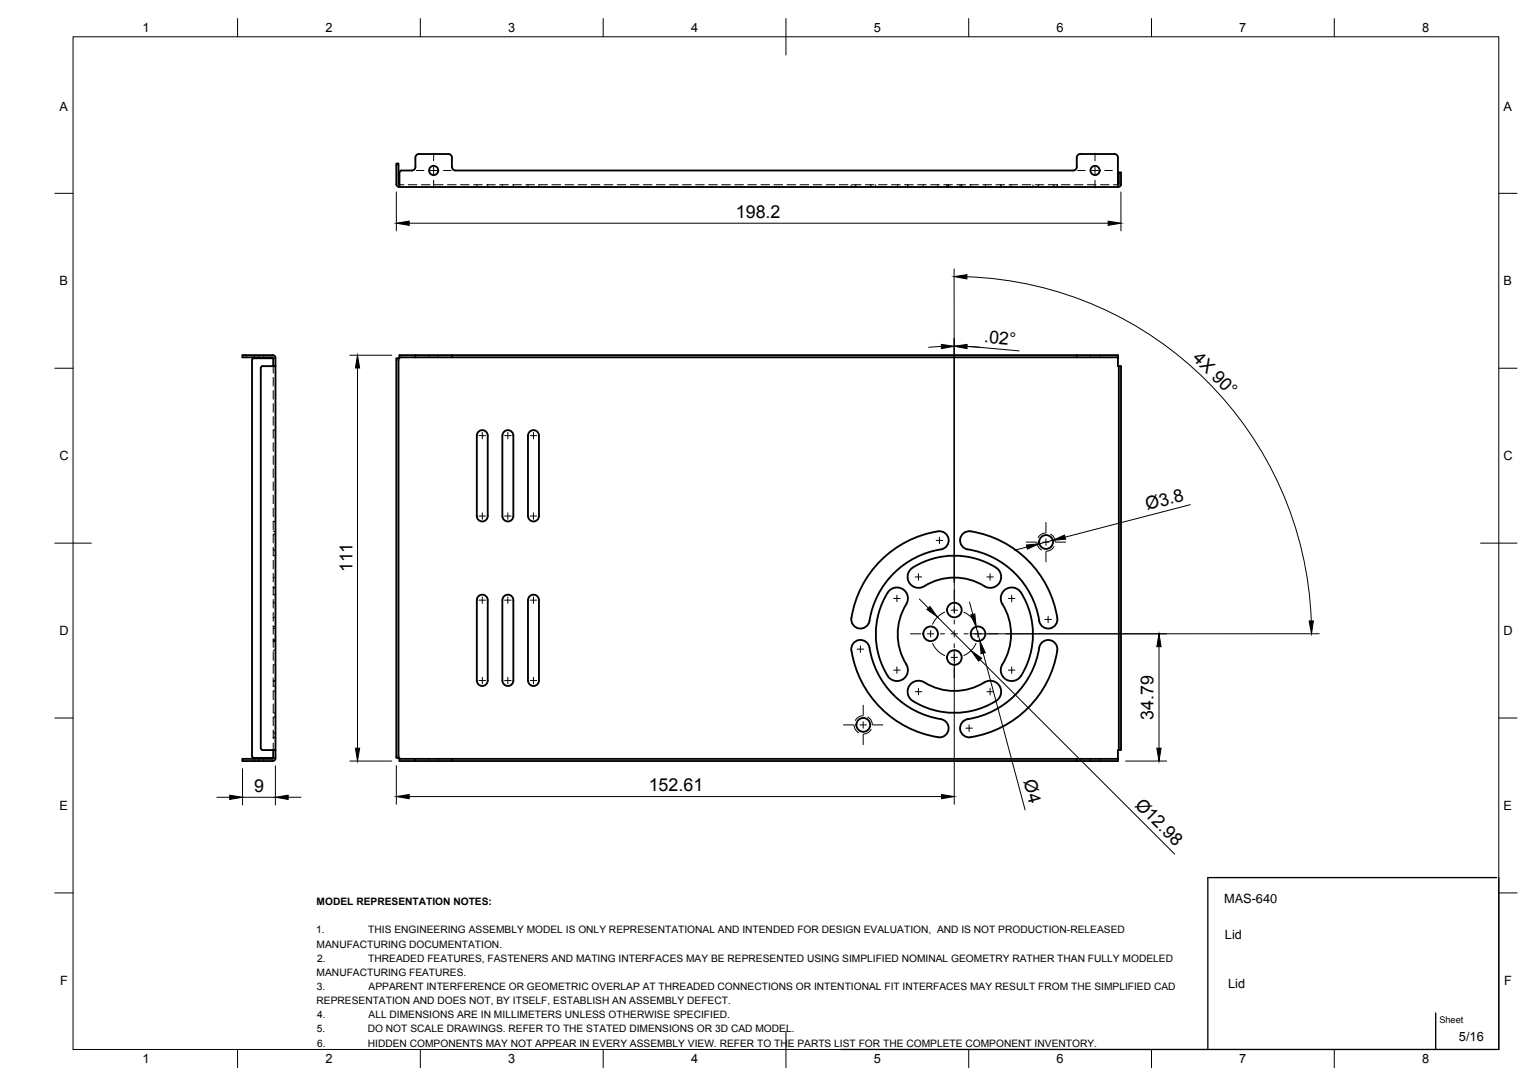
ISO-10303-21;
HEADER;
FILE_DESCRIPTION((''),'2;1');
FILE_NAME('Lid.step','2026-10-09T10:33:02-07:00',(''),(''),'','','');
FILE_SCHEMA (('AUTOMOTIVE_DESIGN { 1 0 10303 214 3 1 1 }'));
ENDSEC;
DATA;
#10=MECHANICAL_DESIGN_GEOMETRIC_PRESENTATION_REPRESENTATION('',(#838),#86330);
#814=SHAPE_REPRESENTATION_RELATIONSHIP('SRR','None',#86453,#826) ;
#826=ADVANCED_BREP_SHAPE_REPRESENTATION('',(#850),#86307) ;
#838=STYLED_ITEM('',(#86581),#850) ;
#850=MANIFOLD_SOLID_BREP('Body1',#32637) ;
#862=CONICAL_SURFACE('',#33010,2.390165042945,0.785398163397448) ;
#863=CONICAL_SURFACE('',#33011,2.390165042945,0.785398163397448) ;
#903=B_SPLINE_SURFACE_WITH_KNOTS('',3,3,((#46889,#46890,#46891,#46892),
(#46893,#46894,#46895,#46896),(#46897,#46898,#46899,#46900),(#46901,#46902,
#46903,#46904),(#46905,#46906,#46907,#46908),(#46909,#46910,#46911,#46912),
(#46913,#46914,#46915,#46916)),.UNSPECIFIED.,.F.,.F.,.F.,(4,1,1,1,4),(4,
4),(0.,0.285714285714286,0.571428571428571,0.857142857142857,1.),(0.250000208289045,
0.310000208302026),.UNSPECIFIED.) ;
#904=B_SPLINE_SURFACE_WITH_KNOTS('',3,3,((#46923,#46924,#46925,#46926),
(#46927,#46928,#46929,#46930),(#46931,#46932,#46933,#46934),(#46935,#46936,
#46937,#46938),(#46939,#46940,#46941,#46942),(#46943,#46944,#46945,#46946),
(#46947,#46948,#46949,#46950)),.UNSPECIFIED.,.F.,.F.,.F.,(4,1,1,1,4),(4,
4),(0.,0.285714285714286,0.571428571428571,0.857142857142857,1.),(-1.50824147057263E-10,
0.0600000000000031),.UNSPECIFIED.) ;
#1000=FACE_BOUND('',#4160,.T.) ;
#1001=FACE_BOUND('',#4161,.T.) ;
#1002=FACE_BOUND('',#4162,.T.) ;
#1003=FACE_BOUND('',#4163,.T.) ;
#1004=FACE_BOUND('',#4164,.T.) ;
#1005=FACE_BOUND('',#4165,.T.) ;
#1006=FACE_BOUND('',#4166,.T.) ;
#1007=FACE_BOUND('',#4167,.T.) ;
#1008=FACE_BOUND('',#4168,.T.) ;
#1009=FACE_BOUND('',#4169,.T.) ;
#1010=FACE_BOUND('',#4170,.T.) ;
#1011=FACE_BOUND('',#4171,.T.) ;
#1012=FACE_BOUND('',#4172,.T.) ;
#1013=FACE_BOUND('',#4173,.T.) ;
#1014=FACE_BOUND('',#4174,.T.) ;
#1015=FACE_BOUND('',#4175,.T.) ;
#1016=FACE_BOUND('',#4176,.T.) ;
#1017=FACE_BOUND('',#4177,.T.) ;
#1018=FACE_BOUND('',#4178,.T.) ;
#1019=FACE_BOUND('',#4179,.T.) ;
#1020=FACE_BOUND('',#4183,.T.) ;
#1021=FACE_BOUND('',#4184,.T.) ;
#1022=FACE_BOUND('',#4188,.T.) ;
#1023=FACE_BOUND('',#4189,.T.) ;
#1024=FACE_BOUND('',#4193,.T.) ;
#1025=FACE_BOUND('',#4194,.T.) ;
#1026=FACE_BOUND('',#4202,.T.) ;
#1027=FACE_BOUND('',#4203,.T.) ;
#1028=FACE_BOUND('',#4204,.T.) ;
#1029=FACE_BOUND('',#4205,.T.) ;
#1030=FACE_BOUND('',#4206,.T.) ;
#1031=FACE_BOUND('',#4207,.T.) ;
#1032=FACE_BOUND('',#4208,.T.) ;
#1033=FACE_BOUND('',#4209,.T.) ;
#1034=FACE_BOUND('',#4210,.T.) ;
#1035=FACE_BOUND('',#4211,.T.) ;
#1036=FACE_BOUND('',#4212,.T.) ;
#1037=FACE_BOUND('',#4213,.T.) ;
#1038=FACE_BOUND('',#4214,.T.) ;
#1039=FACE_BOUND('',#4215,.T.) ;
#1040=FACE_BOUND('',#4216,.T.) ;
#1041=FACE_BOUND('',#4217,.T.) ;
#1042=FACE_BOUND('',#4218,.T.) ;
#1043=FACE_BOUND('',#4219,.T.) ;
#1044=FACE_BOUND('',#4220,.T.) ;
#1045=FACE_BOUND('',#4221,.T.) ;
#1046=FACE_BOUND('',#4223,.T.) ;
#1047=FACE_BOUND('',#4224,.T.) ;
#1189=B_SPLINE_CURVE_WITH_KNOTS('',3,(#46372,#46373,#46374,#46375,#46376,
#46377,#46378),.UNSPECIFIED.,.F.,.F.,(4,1,1,1,4),(0.,0.112519573127489,
0.337558719382466,0.562597865637444,0.787637011892422),.UNSPECIFIED.) ;
#1190=B_SPLINE_CURVE_WITH_KNOTS('',3,(#46384,#46385,#46386,#46387,#46388,
#46389,#46390),.UNSPECIFIED.,.F.,.F.,(4,1,1,1,4),(0.,0.112518191393291,
0.337554574179873,0.562590956966454,0.787627339753036),.UNSPECIFIED.) ;
#1191=B_SPLINE_CURVE_WITH_KNOTS('',3,(#46817,#46818,#46819,#46820,#46821,
#46822,#46823),.UNSPECIFIED.,.F.,.F.,(4,1,1,1,4),(0.,0.22503638292787,0.45007276585574,
0.675109148783609,0.787627340247544),.UNSPECIFIED.) ;
#1192=B_SPLINE_CURVE_WITH_KNOTS('',3,(#46831,#46832,#46833,#46834,#46835,
#46836,#46837),.UNSPECIFIED.,.F.,.F.,(4,1,1,1,4),(0.,0.225039146153262,
0.450078292306524,0.675117438459786,0.787637011536417),.UNSPECIFIED.) ;
#1706=PLANE('',#32777) ;
#1707=PLANE('',#32832) ;
#1708=PLANE('',#32846) ;
#1709=PLANE('',#32847) ;
#1710=PLANE('',#32861) ;
#1711=PLANE('',#32862) ;
#1712=PLANE('',#32875) ;
#1713=PLANE('',#32877) ;
#1714=PLANE('',#32881) ;
#1715=PLANE('',#32882) ;
#1716=PLANE('',#32931) ;
#1717=PLANE('',#32941) ;
#1718=PLANE('',#32956) ;
#1719=PLANE('',#32959) ;
#1720=PLANE('',#32964) ;
#1721=PLANE('',#32965) ;
#1722=PLANE('',#32969) ;
#1723=PLANE('',#32973) ;
#1724=PLANE('',#32975) ;
#1725=PLANE('',#32977) ;
#1726=PLANE('',#32980) ;
#1727=PLANE('',#32982) ;
#1728=PLANE('',#32985) ;
#1729=PLANE('',#32987) ;
#1730=PLANE('',#32990) ;
#1731=PLANE('',#32992) ;
#1732=PLANE('',#32994) ;
#1733=PLANE('',#32997) ;
#1734=PLANE('',#32999) ;
#1735=PLANE('',#33000) ;
#1736=PLANE('',#33003) ;
#1737=PLANE('',#33012) ;
#1738=PLANE('',#33013) ;
#1739=PLANE('',#33019) ;
#1740=PLANE('',#33021) ;
#1741=PLANE('',#33023) ;
#1742=PLANE('',#33025) ;
#1743=PLANE('',#33027) ;
#1744=PLANE('',#33029) ;
#1745=PLANE('',#33031) ;
#1746=PLANE('',#33033) ;
#1747=PLANE('',#33035) ;
#1748=PLANE('',#33037) ;
#1749=PLANE('',#33039) ;
#1750=PLANE('',#33041) ;
#1751=PLANE('',#33043) ;
#2270=FACE_OUTER_BOUND('',#4158,.T.) ;
#2271=FACE_OUTER_BOUND('',#4159,.T.) ;
#2272=FACE_OUTER_BOUND('',#4180,.T.) ;
#2273=FACE_OUTER_BOUND('',#4181,.T.) ;
#2274=FACE_OUTER_BOUND('',#4182,.T.) ;
#2275=FACE_OUTER_BOUND('',#4185,.T.) ;
#2276=FACE_OUTER_BOUND('',#4186,.T.) ;
#2277=FACE_OUTER_BOUND('',#4187,.T.) ;
#2278=FACE_OUTER_BOUND('',#4190,.T.) ;
#2279=FACE_OUTER_BOUND('',#4191,.T.) ;
#2280=FACE_OUTER_BOUND('',#4192,.T.) ;
#2281=FACE_OUTER_BOUND('',#4195,.T.) ;
#2282=FACE_OUTER_BOUND('',#4196,.T.) ;
#2283=FACE_OUTER_BOUND('',#4197,.T.) ;
#2284=FACE_OUTER_BOUND('',#4198,.T.) ;
#2285=FACE_OUTER_BOUND('',#4199,.T.) ;
#2286=FACE_OUTER_BOUND('',#4200,.T.) ;
#2287=FACE_OUTER_BOUND('',#4201,.T.) ;
#2288=FACE_OUTER_BOUND('',#4222,.T.) ;
#2289=FACE_OUTER_BOUND('',#4225,.T.) ;
#2290=FACE_OUTER_BOUND('',#4226,.T.) ;
#2291=FACE_OUTER_BOUND('',#4227,.T.) ;
#2292=FACE_OUTER_BOUND('',#4228,.T.) ;
#2293=FACE_OUTER_BOUND('',#4229,.T.) ;
#2294=FACE_OUTER_BOUND('',#4230,.T.) ;
#2295=FACE_OUTER_BOUND('',#4231,.T.) ;
#2296=FACE_OUTER_BOUND('',#4232,.T.) ;
#2297=FACE_OUTER_BOUND('',#4233,.T.) ;
#2298=FACE_OUTER_BOUND('',#4234,.T.) ;
#2299=FACE_OUTER_BOUND('',#4235,.T.) ;
#2300=FACE_OUTER_BOUND('',#4236,.T.) ;
#2301=FACE_OUTER_BOUND('',#4237,.T.) ;
#2302=FACE_OUTER_BOUND('',#4238,.T.) ;
#2303=FACE_OUTER_BOUND('',#4239,.T.) ;
#2304=FACE_OUTER_BOUND('',#4240,.T.) ;
#2305=FACE_OUTER_BOUND('',#4241,.T.) ;
#2306=FACE_OUTER_BOUND('',#4242,.T.) ;
#2307=FACE_OUTER_BOUND('',#4243,.T.) ;
#2308=FACE_OUTER_BOUND('',#4244,.T.) ;
#2309=FACE_OUTER_BOUND('',#4245,.T.) ;
#2310=FACE_OUTER_BOUND('',#4246,.T.) ;
#2311=FACE_OUTER_BOUND('',#4247,.T.) ;
#2312=FACE_OUTER_BOUND('',#4248,.T.) ;
#2313=FACE_OUTER_BOUND('',#4249,.T.) ;
#2314=FACE_OUTER_BOUND('',#4250,.T.) ;
#2315=FACE_OUTER_BOUND('',#4251,.T.) ;
#2316=FACE_OUTER_BOUND('',#4252,.T.) ;
#2317=FACE_OUTER_BOUND('',#4253,.T.) ;
#2318=FACE_OUTER_BOUND('',#4254,.T.) ;
#2319=FACE_OUTER_BOUND('',#4255,.T.) ;
#2320=FACE_OUTER_BOUND('',#4256,.T.) ;
#2321=FACE_OUTER_BOUND('',#4257,.T.) ;
#2322=FACE_OUTER_BOUND('',#4258,.T.) ;
#2323=FACE_OUTER_BOUND('',#4259,.T.) ;
#2324=FACE_OUTER_BOUND('',#4260,.T.) ;
#2325=FACE_OUTER_BOUND('',#4261,.T.) ;
#2326=FACE_OUTER_BOUND('',#4262,.T.) ;
#2327=FACE_OUTER_BOUND('',#4263,.T.) ;
#2328=FACE_OUTER_BOUND('',#4264,.T.) ;
#2329=FACE_OUTER_BOUND('',#4265,.T.) ;
#2330=FACE_OUTER_BOUND('',#4266,.T.) ;
#2331=FACE_OUTER_BOUND('',#4267,.T.) ;
#2332=FACE_OUTER_BOUND('',#4268,.T.) ;
#2333=FACE_OUTER_BOUND('',#4269,.T.) ;
#2334=FACE_OUTER_BOUND('',#4270,.T.) ;
#2335=FACE_OUTER_BOUND('',#4271,.T.) ;
#2336=FACE_OUTER_BOUND('',#4272,.T.) ;
#2337=FACE_OUTER_BOUND('',#4273,.T.) ;
#2338=FACE_OUTER_BOUND('',#4274,.T.) ;
#2339=FACE_OUTER_BOUND('',#4275,.T.) ;
#2340=FACE_OUTER_BOUND('',#4276,.T.) ;
#2341=FACE_OUTER_BOUND('',#4277,.T.) ;
#2342=FACE_OUTER_BOUND('',#4278,.T.) ;
#2343=FACE_OUTER_BOUND('',#4279,.T.) ;
#2344=FACE_OUTER_BOUND('',#4280,.T.) ;
#2345=FACE_OUTER_BOUND('',#4281,.T.) ;
#2346=FACE_OUTER_BOUND('',#4282,.T.) ;
#2347=FACE_OUTER_BOUND('',#4283,.T.) ;
#2348=FACE_OUTER_BOUND('',#4284,.T.) ;
#2349=FACE_OUTER_BOUND('',#4285,.T.) ;
#2350=FACE_OUTER_BOUND('',#4286,.T.) ;
#2351=FACE_OUTER_BOUND('',#4287,.T.) ;
#2352=FACE_OUTER_BOUND('',#4288,.T.) ;
#2353=FACE_OUTER_BOUND('',#4289,.T.) ;
#2354=FACE_OUTER_BOUND('',#4290,.T.) ;
#2355=FACE_OUTER_BOUND('',#4291,.T.) ;
#2356=FACE_OUTER_BOUND('',#4292,.T.) ;
#2357=FACE_OUTER_BOUND('',#4293,.T.) ;
#2358=FACE_OUTER_BOUND('',#4294,.T.) ;
#2359=FACE_OUTER_BOUND('',#4295,.T.) ;
#2360=FACE_OUTER_BOUND('',#4296,.T.) ;
#2361=FACE_OUTER_BOUND('',#4297,.T.) ;
#2362=FACE_OUTER_BOUND('',#4298,.T.) ;
#2363=FACE_OUTER_BOUND('',#4299,.T.) ;
#2364=FACE_OUTER_BOUND('',#4300,.T.) ;
#2365=FACE_OUTER_BOUND('',#4301,.T.) ;
#2366=FACE_OUTER_BOUND('',#4302,.T.) ;
#2367=FACE_OUTER_BOUND('',#4303,.T.) ;
#2368=FACE_OUTER_BOUND('',#4304,.T.) ;
#2369=FACE_OUTER_BOUND('',#4305,.T.) ;
#2370=FACE_OUTER_BOUND('',#4306,.T.) ;
#2371=FACE_OUTER_BOUND('',#4307,.T.) ;
#2372=FACE_OUTER_BOUND('',#4308,.T.) ;
#2373=FACE_OUTER_BOUND('',#4309,.T.) ;
#2374=FACE_OUTER_BOUND('',#4310,.T.) ;
#2375=FACE_OUTER_BOUND('',#4311,.T.) ;
#2376=FACE_OUTER_BOUND('',#4312,.T.) ;
#2377=FACE_OUTER_BOUND('',#4313,.T.) ;
#2378=FACE_OUTER_BOUND('',#4314,.T.) ;
#2379=FACE_OUTER_BOUND('',#4315,.T.) ;
#2380=FACE_OUTER_BOUND('',#4316,.T.) ;
#2381=FACE_OUTER_BOUND('',#4317,.T.) ;
#2382=FACE_OUTER_BOUND('',#4318,.T.) ;
#2383=FACE_OUTER_BOUND('',#4319,.T.) ;
#2384=FACE_OUTER_BOUND('',#4320,.T.) ;
#2385=FACE_OUTER_BOUND('',#4321,.T.) ;
#2386=FACE_OUTER_BOUND('',#4322,.T.) ;
#2387=FACE_OUTER_BOUND('',#4323,.T.) ;
#2388=FACE_OUTER_BOUND('',#4324,.T.) ;
#2389=FACE_OUTER_BOUND('',#4325,.T.) ;
#2390=FACE_OUTER_BOUND('',#4326,.T.) ;
#2391=FACE_OUTER_BOUND('',#4327,.T.) ;
#2392=FACE_OUTER_BOUND('',#4328,.T.) ;
#2393=FACE_OUTER_BOUND('',#4329,.T.) ;
#2394=FACE_OUTER_BOUND('',#4330,.T.) ;
#2395=FACE_OUTER_BOUND('',#4331,.T.) ;
#2396=FACE_OUTER_BOUND('',#4332,.T.) ;
#2397=FACE_OUTER_BOUND('',#4333,.T.) ;
#4158=EDGE_LOOP('',(#20380,#20381,#20382,#20383)) ;
#4159=EDGE_LOOP('',(#20384,#20385,#20386,#20387,#20388,#20389)) ;
#4160=EDGE_LOOP('',(#20390,#20391,#20392,#20393)) ;
#4161=EDGE_LOOP('',(#20394,#20395,#20396,#20397)) ;
#4162=EDGE_LOOP('',(#20398,#20399,#20400,#20401)) ;
#4163=EDGE_LOOP('',(#20402,#20403,#20404,#20405)) ;
#4164=EDGE_LOOP('',(#20406,#20407,#20408,#20409)) ;
#4165=EDGE_LOOP('',(#20410,#20411,#20412,#20413)) ;
#4166=EDGE_LOOP('',(#20414,#20415,#20416,#20417)) ;
#4167=EDGE_LOOP('',(#20418,#20419,#20420,#20421)) ;
#4168=EDGE_LOOP('',(#20422,#20423,#20424,#20425)) ;
#4169=EDGE_LOOP('',(#20426,#20427,#20428,#20429)) ;
#4170=EDGE_LOOP('',(#20430)) ;
#4171=EDGE_LOOP('',(#20431)) ;
#4172=EDGE_LOOP('',(#20432)) ;
#4173=EDGE_LOOP('',(#20433)) ;
#4174=EDGE_LOOP('',(#20434)) ;
#4175=EDGE_LOOP('',(#20435)) ;
#4176=EDGE_LOOP('',(#20436,#20437,#20438,#20439)) ;
#4177=EDGE_LOOP('',(#20440,#20441,#20442,#20443)) ;
#4178=EDGE_LOOP('',(#20444,#20445,#20446,#20447)) ;
#4179=EDGE_LOOP('',(#20448,#20449,#20450,#20451)) ;
#4180=EDGE_LOOP('',(#20452,#20453,#20454,#20455)) ;
#4181=EDGE_LOOP('',(#20456,#20457,#20458,#20459)) ;
#4182=EDGE_LOOP('',(#20460,#20461,#20462,#20463,#20464,#20465,#20466,#20467,
#20468,#20469,#20470,#20471,#20472,#20473,#20474,#20475,#20476,#20477)) ;
#4183=EDGE_LOOP('',(#20478)) ;
#4184=EDGE_LOOP('',(#20479)) ;
#4185=EDGE_LOOP('',(#20480,#20481,#20482,#20483)) ;
#4186=EDGE_LOOP('',(#20484,#20485,#20486,#20487,#20488,#20489,#20490,#20491)) ;
#4187=EDGE_LOOP('',(#20492,#20493,#20494,#20495,#20496,#20497,#20498,#20499,
#20500,#20501,#20502,#20503,#20504,#20505,#20506,#20507,#20508,#20509)) ;
#4188=EDGE_LOOP('',(#20510)) ;
#4189=EDGE_LOOP('',(#20511)) ;
#4190=EDGE_LOOP('',(#20512,#20513,#20514,#20515)) ;
#4191=EDGE_LOOP('',(#20516,#20517,#20518,#20519,#20520,#20521,#20522)) ;
#4192=EDGE_LOOP('',(#20523,#20524,#20525,#20526,#20527,#20528,#20529,#20530,
#20531,#20532,#20533,#20534,#20535,#20536,#20537,#20538,#20539,#20540)) ;
#4193=EDGE_LOOP('',(#20541)) ;
#4194=EDGE_LOOP('',(#20542)) ;
#4195=EDGE_LOOP('',(#20543,#20544,#20545,#20546)) ;
#4196=EDGE_LOOP('',(#20547,#20548,#20549,#20550)) ;
#4197=EDGE_LOOP('',(#20551,#20552,#20553,#20554)) ;
#4198=EDGE_LOOP('',(#20555,#20556,#20557,#20558)) ;
#4199=EDGE_LOOP('',(#20559,#20560,#20561,#20562)) ;
#4200=EDGE_LOOP('',(#20563,#20564,#20565,#20566,#20567,#20568,#20569)) ;
#4201=EDGE_LOOP('',(#20570,#20571,#20572,#20573,#20574,#20575,#20576,#20577,
#20578,#20579,#20580,#20581)) ;
#4202=EDGE_LOOP('',(#20582,#20583,#20584,#20585)) ;
#4203=EDGE_LOOP('',(#20586)) ;
#4204=EDGE_LOOP('',(#20587)) ;
#4205=EDGE_LOOP('',(#20588,#20589,#20590,#20591)) ;
#4206=EDGE_LOOP('',(#20592,#20593,#20594,#20595)) ;
#4207=EDGE_LOOP('',(#20596,#20597,#20598,#20599)) ;
#4208=EDGE_LOOP('',(#20600,#20601,#20602,#20603)) ;
#4209=EDGE_LOOP('',(#20604,#20605,#20606,#20607)) ;
#4210=EDGE_LOOP('',(#20608,#20609,#20610,#20611)) ;
#4211=EDGE_LOOP('',(#20612)) ;
#4212=EDGE_LOOP('',(#20613)) ;
#4213=EDGE_LOOP('',(#20614)) ;
#4214=EDGE_LOOP('',(#20615)) ;
#4215=EDGE_LOOP('',(#20616,#20617,#20618,#20619)) ;
#4216=EDGE_LOOP('',(#20620,#20621,#20622,#20623)) ;
#4217=EDGE_LOOP('',(#20624,#20625,#20626,#20627)) ;
#4218=EDGE_LOOP('',(#20628,#20629,#20630,#20631)) ;
#4219=EDGE_LOOP('',(#20632,#20633,#20634,#20635)) ;
#4220=EDGE_LOOP('',(#20636,#20637,#20638,#20639)) ;
#4221=EDGE_LOOP('',(#20640,#20641,#20642,#20643)) ;
#4222=EDGE_LOOP('',(#20644,#20645,#20646,#20647,#20648,#20649,#20650,#20651,
#20652,#20653,#20654,#20655,#20656,#20657,#20658,#20659,#20660,#20661)) ;
#4223=EDGE_LOOP('',(#20662)) ;
#4224=EDGE_LOOP('',(#20663)) ;
#4225=EDGE_LOOP('',(#20664,#20665,#20666,#20667,#20668,#20669)) ;
#4226=EDGE_LOOP('',(#20670,#20671,#20672,#20673)) ;
#4227=EDGE_LOOP('',(#20674,#20675,#20676,#20677)) ;
#4228=EDGE_LOOP('',(#20678,#20679,#20680,#20681)) ;
#4229=EDGE_LOOP('',(#20682,#20683,#20684,#20685)) ;
#4230=EDGE_LOOP('',(#20686,#20687,#20688,#20689)) ;
#4231=EDGE_LOOP('',(#20690,#20691,#20692,#20693)) ;
#4232=EDGE_LOOP('',(#20694,#20695,#20696,#20697)) ;
#4233=EDGE_LOOP('',(#20698,#20699,#20700,#20701)) ;
#4234=EDGE_LOOP('',(#20702,#20703,#20704,#20705)) ;
#4235=EDGE_LOOP('',(#20706,#20707,#20708,#20709)) ;
#4236=EDGE_LOOP('',(#20710,#20711,#20712,#20713)) ;
#4237=EDGE_LOOP('',(#20714,#20715,#20716,#20717)) ;
#4238=EDGE_LOOP('',(#20718,#20719,#20720,#20721)) ;
#4239=EDGE_LOOP('',(#20722,#20723,#20724,#20725)) ;
#4240=EDGE_LOOP('',(#20726,#20727,#20728,#20729)) ;
#4241=EDGE_LOOP('',(#20730,#20731,#20732,#20733,#20734,#20735,#20736)) ;
#4242=EDGE_LOOP('',(#20737,#20738,#20739,#20740)) ;
#4243=EDGE_LOOP('',(#20741,#20742,#20743,#20744)) ;
#4244=EDGE_LOOP('',(#20745,#20746,#20747,#20748)) ;
#4245=EDGE_LOOP('',(#20749,#20750,#20751,#20752,#20753,#20754)) ;
#4246=EDGE_LOOP('',(#20755,#20756,#20757,#20758)) ;
#4247=EDGE_LOOP('',(#20759,#20760,#20761,#20762,#20763,#20764,#20765)) ;
#4248=EDGE_LOOP('',(#20766,#20767,#20768,#20769)) ;
#4249=EDGE_LOOP('',(#20770,#20771,#20772,#20773,#20774,#20775,#20776)) ;
#4250=EDGE_LOOP('',(#20777,#20778,#20779,#20780)) ;
#4251=EDGE_LOOP('',(#20781,#20782,#20783,#20784)) ;
#4252=EDGE_LOOP('',(#20785,#20786,#20787,#20788)) ;
#4253=EDGE_LOOP('',(#20789,#20790,#20791,#20792)) ;
#4254=EDGE_LOOP('',(#20793,#20794,#20795,#20796)) ;
#4255=EDGE_LOOP('',(#20797,#20798,#20799,#20800)) ;
#4256=EDGE_LOOP('',(#20801,#20802,#20803,#20804)) ;
#4257=EDGE_LOOP('',(#20805,#20806,#20807,#20808)) ;
#4258=EDGE_LOOP('',(#20809,#20810,#20811,#20812)) ;
#4259=EDGE_LOOP('',(#20813,#20814,#20815,#20816)) ;
#4260=EDGE_LOOP('',(#20817,#20818,#20819,#20820)) ;
#4261=EDGE_LOOP('',(#20821,#20822,#20823,#20824)) ;
#4262=EDGE_LOOP('',(#20825,#20826,#20827,#20828)) ;
#4263=EDGE_LOOP('',(#20829,#20830,#20831,#20832)) ;
#4264=EDGE_LOOP('',(#20833,#20834,#20835,#20836)) ;
#4265=EDGE_LOOP('',(#20837,#20838,#20839,#20840)) ;
#4266=EDGE_LOOP('',(#20841,#20842,#20843,#20844)) ;
#4267=EDGE_LOOP('',(#20845,#20846,#20847,#20848)) ;
#4268=EDGE_LOOP('',(#20849,#20850,#20851,#20852)) ;
#4269=EDGE_LOOP('',(#20853,#20854,#20855,#20856)) ;
#4270=EDGE_LOOP('',(#20857,#20858,#20859,#20860)) ;
#4271=EDGE_LOOP('',(#20861,#20862,#20863,#20864)) ;
#4272=EDGE_LOOP('',(#20865,#20866,#20867,#20868,#20869,#20870,#20871)) ;
#4273=EDGE_LOOP('',(#20872,#20873,#20874,#20875,#20876,#20877,#20878,#20879)) ;
#4274=EDGE_LOOP('',(#20880,#20881,#20882,#20883)) ;
#4275=EDGE_LOOP('',(#20884,#20885,#20886,#20887)) ;
#4276=EDGE_LOOP('',(#20888,#20889,#20890,#20891)) ;
#4277=EDGE_LOOP('',(#20892,#20893,#20894,#20895)) ;
#4278=EDGE_LOOP('',(#20896,#20897,#20898,#20899)) ;
#4279=EDGE_LOOP('',(#20900,#20901,#20902,#20903)) ;
#4280=EDGE_LOOP('',(#20904,#20905,#20906,#20907)) ;
#4281=EDGE_LOOP('',(#20908,#20909,#20910,#20911)) ;
#4282=EDGE_LOOP('',(#20912,#20913,#20914,#20915)) ;
#4283=EDGE_LOOP('',(#20916,#20917,#20918,#20919)) ;
#4284=EDGE_LOOP('',(#20920,#20921,#20922,#20923)) ;
#4285=EDGE_LOOP('',(#20924,#20925,#20926,#20927)) ;
#4286=EDGE_LOOP('',(#20928,#20929,#20930,#20931)) ;
#4287=EDGE_LOOP('',(#20932,#20933,#20934,#20935,#20936,#20937)) ;
#4288=EDGE_LOOP('',(#20938,#20939,#20940,#20941)) ;
#4289=EDGE_LOOP('',(#20942,#20943,#20944,#20945)) ;
#4290=EDGE_LOOP('',(#20946,#20947,#20948,#20949)) ;
#4291=EDGE_LOOP('',(#20950,#20951,#20952,#20953)) ;
#4292=EDGE_LOOP('',(#20954,#20955,#20956,#20957)) ;
#4293=EDGE_LOOP('',(#20958,#20959,#20960,#20961)) ;
#4294=EDGE_LOOP('',(#20962,#20963,#20964,#20965)) ;
#4295=EDGE_LOOP('',(#20966,#20967,#20968,#20969)) ;
#4296=EDGE_LOOP('',(#20970,#20971,#20972,#20973)) ;
#4297=EDGE_LOOP('',(#20974,#20975,#20976,#20977)) ;
#4298=EDGE_LOOP('',(#20978,#20979,#20980,#20981)) ;
#4299=EDGE_LOOP('',(#20982,#20983,#20984,#20985)) ;
#4300=EDGE_LOOP('',(#20986,#20987,#20988,#20989)) ;
#4301=EDGE_LOOP('',(#20990,#20991,#20992,#20993)) ;
#4302=EDGE_LOOP('',(#20994,#20995,#20996,#20997)) ;
#4303=EDGE_LOOP('',(#20998,#20999,#21000,#21001)) ;
#4304=EDGE_LOOP('',(#21002,#21003,#21004,#21005)) ;
#4305=EDGE_LOOP('',(#21006,#21007,#21008,#21009)) ;
#4306=EDGE_LOOP('',(#21010,#21011,#21012,#21013)) ;
#4307=EDGE_LOOP('',(#21014,#21015,#21016,#21017)) ;
#4308=EDGE_LOOP('',(#21018,#21019,#21020,#21021)) ;
#4309=EDGE_LOOP('',(#21022,#21023,#21024,#21025)) ;
#4310=EDGE_LOOP('',(#21026,#21027,#21028,#21029)) ;
#4311=EDGE_LOOP('',(#21030,#21031,#21032,#21033)) ;
#4312=EDGE_LOOP('',(#21034,#21035,#21036,#21037)) ;
#4313=EDGE_LOOP('',(#21038,#21039,#21040,#21041)) ;
#4314=EDGE_LOOP('',(#21042,#21043,#21044,#21045)) ;
#4315=EDGE_LOOP('',(#21046,#21047,#21048,#21049)) ;
#4316=EDGE_LOOP('',(#21050,#21051,#21052,#21053)) ;
#4317=EDGE_LOOP('',(#21054,#21055,#21056,#21057,#21058,#21059)) ;
#4318=EDGE_LOOP('',(#21060,#21061,#21062,#21063)) ;
#4319=EDGE_LOOP('',(#21064,#21065,#21066,#21067)) ;
#4320=EDGE_LOOP('',(#21068,#21069,#21070,#21071)) ;
#4321=EDGE_LOOP('',(#21072,#21073,#21074,#21075)) ;
#4322=EDGE_LOOP('',(#21076,#21077,#21078,#21079)) ;
#4323=EDGE_LOOP('',(#21080,#21081,#21082,#21083)) ;
#4324=EDGE_LOOP('',(#21084,#21085,#21086,#21087)) ;
#4325=EDGE_LOOP('',(#21088,#21089,#21090,#21091)) ;
#4326=EDGE_LOOP('',(#21092,#21093,#21094,#21095)) ;
#4327=EDGE_LOOP('',(#21096,#21097,#21098,#21099)) ;
#4328=EDGE_LOOP('',(#21100,#21101,#21102,#21103)) ;
#4329=EDGE_LOOP('',(#21104,#21105,#21106,#21107)) ;
#4330=EDGE_LOOP('',(#21108,#21109,#21110,#21111)) ;
#4331=EDGE_LOOP('',(#21112,#21113,#21114,#21115)) ;
#4332=EDGE_LOOP('',(#21116,#21117,#21118,#21119)) ;
#4333=EDGE_LOOP('',(#21120,#21121,#21122,#21123)) ;
#6235=LINE('',#46354,#8554) ;
#6236=LINE('',#46357,#8555) ;
#6237=LINE('',#46360,#8556) ;
#6238=LINE('',#46362,#8557) ;
#6239=LINE('',#46364,#8558) ;
#6240=LINE('',#46366,#8559) ;
#6241=LINE('',#46367,#8560) ;
#6242=LINE('',#46414,#8561) ;
#6243=LINE('',#46418,#8562) ;
#6244=LINE('',#46422,#8563) ;
#6245=LINE('',#46426,#8564) ;
#6246=LINE('',#46430,#8565) ;
#6247=LINE('',#46434,#8566) ;
#6248=LINE('',#46438,#8567) ;
#6249=LINE('',#46442,#8568) ;
#6250=LINE('',#46446,#8569) ;
#6251=LINE('',#46450,#8570) ;
#6252=LINE('',#46454,#8571) ;
#6253=LINE('',#46458,#8572) ;
#6254=LINE('',#46509,#8573) ;
#6255=LINE('',#46514,#8574) ;
#6256=LINE('',#46518,#8575) ;
#6257=LINE('',#46522,#8576) ;
#6258=LINE('',#46526,#8577) ;
#6259=LINE('',#46530,#8578) ;
#6260=LINE('',#46534,#8579) ;
#6261=LINE('',#46538,#8580) ;
#6262=LINE('',#46542,#8581) ;
#6263=LINE('',#46546,#8582) ;
#6264=LINE('',#46549,#8583) ;
#6265=LINE('',#46559,#8584) ;
#6266=LINE('',#46562,#8585) ;
#6267=LINE('',#46565,#8586) ;
#6268=LINE('',#46567,#8587) ;
#6269=LINE('',#46568,#8588) ;
#6270=LINE('',#46570,#8589) ;
#6271=LINE('',#46571,#8590) ;
#6272=LINE('',#46574,#8591) ;
#6273=LINE('',#46578,#8592) ;
#6274=LINE('',#46582,#8593) ;
#6275=LINE('',#46586,#8594) ;
#6276=LINE('',#46590,#8595) ;
#6277=LINE('',#46594,#8596) ;
#6278=LINE('',#46598,#8597) ;
#6279=LINE('',#46602,#8598) ;
#6280=LINE('',#46613,#8599) ;
#6281=LINE('',#46616,#8600) ;
#6282=LINE('',#46619,#8601) ;
#6283=LINE('',#46620,#8602) ;
#6284=LINE('',#46622,#8603) ;
#6285=LINE('',#46623,#8604) ;
#6286=LINE('',#46626,#8605) ;
#6287=LINE('',#46630,#8606) ;
#6288=LINE('',#46634,#8607) ;
#6289=LINE('',#46638,#8608) ;
#6290=LINE('',#46642,#8609) ;
#6291=LINE('',#46646,#8610) ;
#6292=LINE('',#46650,#8611) ;
#6293=LINE('',#46654,#8612) ;
#6294=LINE('',#46662,#8613) ;
#6295=LINE('',#46665,#8614) ;
#6296=LINE('',#46668,#8615) ;
#6297=LINE('',#46669,#8616) ;
#6298=LINE('',#46671,#8617) ;
#6299=LINE('',#46672,#8618) ;
#6300=LINE('',#46674,#8619) ;
#6301=LINE('',#46680,#8620) ;
#6302=LINE('',#46683,#8621) ;
#6303=LINE('',#46685,#8622) ;
#6304=LINE('',#46687,#8623) ;
#6305=LINE('',#46689,#8624) ;
#6306=LINE('',#46690,#8625) ;
#6307=LINE('',#46693,#8626) ;
#6308=LINE('',#46694,#8627) ;
#6309=LINE('',#46696,#8628) ;
#6310=LINE('',#46698,#8629) ;
#6311=LINE('',#46700,#8630) ;
#6312=LINE('',#46701,#8631) ;
#6313=LINE('',#46718,#8632) ;
#6314=LINE('',#46721,#8633) ;
#6315=LINE('',#46726,#8634) ;
#6316=LINE('',#46729,#8635) ;
#6317=LINE('',#46734,#8636) ;
#6318=LINE('',#46737,#8637) ;
#6319=LINE('',#46742,#8638) ;
#6320=LINE('',#46745,#8639) ;
#6321=LINE('',#46750,#8640) ;
#6322=LINE('',#46753,#8641) ;
#6323=LINE('',#46758,#8642) ;
#6324=LINE('',#46761,#8643) ;
#6325=LINE('',#46842,#8644) ;
#6326=LINE('',#46846,#8645) ;
#6327=LINE('',#46850,#8646) ;
#6328=LINE('',#46854,#8647) ;
#6329=LINE('',#46858,#8648) ;
#6330=LINE('',#46861,#8649) ;
#6331=LINE('',#46864,#8650) ;
#6332=LINE('',#46871,#8651) ;
#6333=LINE('',#46875,#8652) ;
#6334=LINE('',#46878,#8653) ;
#6335=LINE('',#46879,#8654) ;
#6336=LINE('',#46881,#8655) ;
#6337=LINE('',#46883,#8656) ;
#6338=LINE('',#46884,#8657) ;
#6339=LINE('',#46886,#8658) ;
#6340=LINE('',#46888,#8659) ;
#6341=LINE('',#46917,#8660) ;
#6342=LINE('',#46918,#8661) ;
#6343=LINE('',#46920,#8662) ;
#6344=LINE('',#46922,#8663) ;
#6345=LINE('',#46951,#8664) ;
#6346=LINE('',#46952,#8665) ;
#6347=LINE('',#46954,#8666) ;
#6348=LINE('',#46956,#8667) ;
#6349=LINE('',#46958,#8668) ;
#6350=LINE('',#46961,#8669) ;
#6351=LINE('',#46965,#8670) ;
#6352=LINE('',#46966,#8671) ;
#6353=LINE('',#46969,#8672) ;
#6354=LINE('',#46972,#8673) ;
#6355=LINE('',#46973,#8674) ;
#6356=LINE('',#46980,#8675) ;
#6357=LINE('',#46983,#8676) ;
#6358=LINE('',#46986,#8677) ;
#6359=LINE('',#46988,#8678) ;
#6360=LINE('',#46989,#8679) ;
#6361=LINE('',#46992,#8680) ;
#6362=LINE('',#46994,#8681) ;
#6363=LINE('',#46996,#8682) ;
#6364=LINE('',#47001,#8683) ;
#6365=LINE('',#47005,#8684) ;
#6366=LINE('',#47007,#8685) ;
#6367=LINE('',#47009,#8686) ;
#6368=LINE('',#47012,#8687) ;
#6369=LINE('',#47013,#8688) ;
#6370=LINE('',#47015,#8689) ;
#6371=LINE('',#47017,#8690) ;
#6372=LINE('',#47018,#8691) ;
#6373=LINE('',#47020,#8692) ;
#6374=LINE('',#47023,#8693) ;
#6375=LINE('',#47024,#8694) ;
#6376=LINE('',#47026,#8695) ;
#6377=LINE('',#47028,#8696) ;
#6378=LINE('',#47029,#8697) ;
#6379=LINE('',#47032,#8698) ;
#6380=LINE('',#47034,#8699) ;
#6381=LINE('',#47035,#8700) ;
#6382=LINE('',#47037,#8701) ;
#6383=LINE('',#47039,#8702) ;
#6384=LINE('',#47041,#8703) ;
#6385=LINE('',#47044,#8704) ;
#6386=LINE('',#47045,#8705) ;
#6387=LINE('',#47047,#8706) ;
#6388=LINE('',#47049,#8707) ;
#6389=LINE('',#47051,#8708) ;
#6390=LINE('',#47053,#8709) ;
#6391=LINE('',#47059,#8710) ;
#6392=LINE('',#47064,#8711) ;
#6393=LINE('',#47066,#8712) ;
#6394=LINE('',#47069,#8713) ;
#6395=LINE('',#47071,#8714) ;
#6396=LINE('',#47072,#8715) ;
#6397=LINE('',#47074,#8716) ;
#6398=LINE('',#47075,#8717) ;
#6399=LINE('',#47080,#8718) ;
#6400=LINE('',#47082,#8719) ;
#6401=LINE('',#47086,#8720) ;
#6402=LINE('',#47088,#8721) ;
#6403=LINE('',#47090,#8722) ;
#6404=LINE('',#47092,#8723) ;
#6405=LINE('',#47094,#8724) ;
#6406=LINE('',#47095,#8725) ;
#6407=LINE('',#47097,#8726) ;
#6408=LINE('',#47099,#8727) ;
#6409=LINE('',#47102,#8728) ;
#6410=LINE('',#47103,#8729) ;
#6411=LINE('',#47105,#8730) ;
#6412=LINE('',#47107,#8731) ;
#6413=LINE('',#47110,#8732) ;
#6414=LINE('',#47111,#8733) ;
#6415=LINE('',#47113,#8734) ;
#6416=LINE('',#47115,#8735) ;
#6417=LINE('',#47118,#8736) ;
#6418=LINE('',#47119,#8737) ;
#6419=LINE('',#47121,#8738) ;
#6420=LINE('',#47123,#8739) ;
#6421=LINE('',#47126,#8740) ;
#6422=LINE('',#47127,#8741) ;
#6423=LINE('',#47129,#8742) ;
#6424=LINE('',#47131,#8743) ;
#6425=LINE('',#47134,#8744) ;
#6426=LINE('',#47135,#8745) ;
#6427=LINE('',#47137,#8746) ;
#6428=LINE('',#47139,#8747) ;
#6429=LINE('',#47142,#8748) ;
#6430=LINE('',#47145,#8749) ;
#6431=LINE('',#47150,#8750) ;
#6432=LINE('',#47151,#8751) ;
#6433=LINE('',#47153,#8752) ;
#6434=LINE('',#47154,#8753) ;
#6435=LINE('',#47158,#8754) ;
#6436=LINE('',#47159,#8755) ;
#6437=LINE('',#47161,#8756) ;
#6438=LINE('',#47162,#8757) ;
#6439=LINE('',#47166,#8758) ;
#6440=LINE('',#47167,#8759) ;
#6441=LINE('',#47169,#8760) ;
#6442=LINE('',#47170,#8761) ;
#8554=VECTOR('',#36533,10.) ;
#8555=VECTOR('',#36536,10.) ;
#8556=VECTOR('',#36539,10.) ;
#8557=VECTOR('',#36540,10.) ;
#8558=VECTOR('',#36541,10.) ;
#8559=VECTOR('',#36542,10.) ;
#8560=VECTOR('',#36543,10.) ;
#8561=VECTOR('',#36572,10.) ;
#8562=VECTOR('',#36575,10.) ;
#8563=VECTOR('',#36578,10.) ;
#8564=VECTOR('',#36581,10.) ;
#8565=VECTOR('',#36584,10.) ;
#8566=VECTOR('',#36587,10.) ;
#8567=VECTOR('',#36590,10.) ;
#8568=VECTOR('',#36593,10.) ;
#8569=VECTOR('',#36596,10.) ;
#8570=VECTOR('',#36599,10.) ;
#8571=VECTOR('',#36602,10.) ;
#8572=VECTOR('',#36605,10.) ;
#8573=VECTOR('',#36658,10.) ;
#8574=VECTOR('',#36663,10.) ;
#8575=VECTOR('',#36668,10.) ;
#8576=VECTOR('',#36671,10.) ;
#8577=VECTOR('',#36674,10.) ;
#8578=VECTOR('',#36677,10.) ;
#8579=VECTOR('',#36680,10.) ;
#8580=VECTOR('',#36683,10.) ;
#8581=VECTOR('',#36686,10.) ;
#8582=VECTOR('',#36689,10.) ;
#8583=VECTOR('',#36692,10.) ;
#8584=VECTOR('',#36701,10.) ;
#8585=VECTOR('',#36704,10.) ;
#8586=VECTOR('',#36707,10.) ;
#8587=VECTOR('',#36708,10.) ;
#8588=VECTOR('',#36709,10.) ;
#8589=VECTOR('',#36710,10.) ;
#8590=VECTOR('',#36711,10.) ;
#8591=VECTOR('',#36714,10.) ;
#8592=VECTOR('',#36717,10.) ;
#8593=VECTOR('',#36720,10.) ;
#8594=VECTOR('',#36723,10.) ;
#8595=VECTOR('',#36726,10.) ;
#8596=VECTOR('',#36729,10.) ;
#8597=VECTOR('',#36732,10.) ;
#8598=VECTOR('',#36735,10.) ;
#8599=VECTOR('',#36746,10.) ;
#8600=VECTOR('',#36749,10.) ;
#8601=VECTOR('',#36752,10.) ;
#8602=VECTOR('',#36753,10.) ;
#8603=VECTOR('',#36754,1.711483519287) ;
#8604=VECTOR('',#36755,10.) ;
#8605=VECTOR('',#36758,10.) ;
#8606=VECTOR('',#36761,10.) ;
#8607=VECTOR('',#36764,10.) ;
#8608=VECTOR('',#36767,10.) ;
#8609=VECTOR('',#36770,10.) ;
#8610=VECTOR('',#36773,10.) ;
#8611=VECTOR('',#36776,10.) ;
#8612=VECTOR('',#36779,10.) ;
#8613=VECTOR('',#36788,10.) ;
#8614=VECTOR('',#36791,10.) ;
#8615=VECTOR('',#36794,10.) ;
#8616=VECTOR('',#36795,10.) ;
#8617=VECTOR('',#36798,10.) ;
#8618=VECTOR('',#36799,10.) ;
#8619=VECTOR('',#36802,10.) ;
#8620=VECTOR('',#36807,10.) ;
#8621=VECTOR('',#36810,10.) ;
#8622=VECTOR('',#36813,10.) ;
#8623=VECTOR('',#36814,10.) ;
#8624=VECTOR('',#36815,10.) ;
#8625=VECTOR('',#36816,10.) ;
#8626=VECTOR('',#36819,10.) ;
#8627=VECTOR('',#36820,0.1) ;
#8628=VECTOR('',#36821,0.09999999999997) ;
#8629=VECTOR('',#36822,108.3) ;
#8630=VECTOR('',#36823,0.09999999999997) ;
#8631=VECTOR('',#36824,0.1) ;
#8632=VECTOR('',#36839,22.) ;
#8633=VECTOR('',#36842,22.) ;
#8634=VECTOR('',#36845,22.) ;
#8635=VECTOR('',#36848,22.) ;
#8636=VECTOR('',#36851,22.) ;
#8637=VECTOR('',#36854,22.) ;
#8638=VECTOR('',#36857,22.) ;
#8639=VECTOR('',#36860,22.) ;
#8640=VECTOR('',#36863,22.) ;
#8641=VECTOR('',#36866,22.) ;
#8642=VECTOR('',#36869,22.) ;
#8643=VECTOR('',#36872,22.) ;
#8644=VECTOR('',#36937,10.) ;
#8645=VECTOR('',#36940,10.) ;
#8646=VECTOR('',#36943,10.) ;
#8647=VECTOR('',#36946,10.) ;
#8648=VECTOR('',#36949,10.) ;
#8649=VECTOR('',#36952,10.) ;
#8650=VECTOR('',#36955,10.) ;
#8651=VECTOR('',#36962,10.) ;
#8652=VECTOR('',#36965,10.) ;
#8653=VECTOR('',#36970,10.) ;
#8654=VECTOR('',#36971,0.75) ;
#8655=VECTOR('',#36974,10.) ;
#8656=VECTOR('',#36977,10.) ;
#8657=VECTOR('',#36978,10.) ;
#8658=VECTOR('',#36981,10.) ;
#8659=VECTOR('',#36984,0.75) ;
#8660=VECTOR('',#36985,10.) ;
#8661=VECTOR('',#36986,10.) ;
#8662=VECTOR('',#36989,10.) ;
#8663=VECTOR('',#36992,0.75) ;
#8664=VECTOR('',#36993,10.) ;
#8665=VECTOR('',#36994,0.7499999999999) ;
#8666=VECTOR('',#36997,10.) ;
#8667=VECTOR('',#37000,0.75) ;
#8668=VECTOR('',#37003,0.7499999999999) ;
#8669=VECTOR('',#37006,10.) ;
#8670=VECTOR('',#37011,10.) ;
#8671=VECTOR('',#37012,10.) ;
#8672=VECTOR('',#37015,10.) ;
#8673=VECTOR('',#37020,10.) ;
#8674=VECTOR('',#37021,10.) ;
#8675=VECTOR('',#37028,10.) ;
#8676=VECTOR('',#37031,10.) ;
#8677=VECTOR('',#37034,10.) ;
#8678=VECTOR('',#37035,10.) ;
#8679=VECTOR('',#37036,10.) ;
#8680=VECTOR('',#37039,10.) ;
#8681=VECTOR('',#37040,10.) ;
#8682=VECTOR('',#37041,10.) ;
#8683=VECTOR('',#37048,10.) ;
#8684=VECTOR('',#37053,5.5) ;
#8685=VECTOR('',#37056,10.) ;
#8686=VECTOR('',#37059,10.) ;
#8687=VECTOR('',#37064,10.) ;
#8688=VECTOR('',#37065,10.) ;
#8689=VECTOR('',#37068,10.) ;
#8690=VECTOR('',#37071,10.) ;
#8691=VECTOR('',#37072,10.) ;
#8692=VECTOR('',#37075,10.) ;
#8693=VECTOR('',#37080,10.) ;
#8694=VECTOR('',#37081,10.) ;
#8695=VECTOR('',#37084,10.) ;
#8696=VECTOR('',#37087,10.) ;
#8697=VECTOR('',#37088,10.) ;
#8698=VECTOR('',#37093,10.) ;
#8699=VECTOR('',#37096,10.) ;
#8700=VECTOR('',#37097,10.) ;
#8701=VECTOR('',#37100,10.) ;
#8702=VECTOR('',#37103,10.) ;
#8703=VECTOR('',#37106,10.) ;
#8704=VECTOR('',#37111,10.) ;
#8705=VECTOR('',#37112,10.) ;
#8706=VECTOR('',#37115,10.) ;
#8707=VECTOR('',#37118,10.) ;
#8708=VECTOR('',#37121,10.) ;
#8709=VECTOR('',#37124,10.) ;
#8710=VECTOR('',#37133,5.5) ;
#8711=VECTOR('',#37142,1.25) ;
#8712=VECTOR('',#37145,1.25) ;
#8713=VECTOR('',#37150,1.25) ;
#8714=VECTOR('',#37153,0.75) ;
#8715=VECTOR('',#37154,0.75) ;
#8716=VECTOR('',#37157,0.75) ;
#8717=VECTOR('',#37158,0.75) ;
#8718=VECTOR('',#37167,2.390165042945) ;
#8719=VECTOR('',#37170,2.390165042945) ;
#8720=VECTOR('',#37177,2.) ;
#8721=VECTOR('',#37180,2.) ;
#8722=VECTOR('',#37183,2.) ;
#8723=VECTOR('',#37186,2.) ;
#8724=VECTOR('',#37189,0.75) ;
#8725=VECTOR('',#37190,0.75) ;
#8726=VECTOR('',#37193,0.75) ;
#8727=VECTOR('',#37196,0.75) ;
#8728=VECTOR('',#37201,0.75) ;
#8729=VECTOR('',#37202,0.75) ;
#8730=VECTOR('',#37205,0.75) ;
#8731=VECTOR('',#37208,0.75) ;
#8732=VECTOR('',#37213,0.75) ;
#8733=VECTOR('',#37214,0.75) ;
#8734=VECTOR('',#37217,0.75) ;
#8735=VECTOR('',#37220,0.75) ;
#8736=VECTOR('',#37225,0.75) ;
#8737=VECTOR('',#37226,0.75) ;
#8738=VECTOR('',#37229,0.75) ;
#8739=VECTOR('',#37232,0.75) ;
#8740=VECTOR('',#37237,0.75) ;
#8741=VECTOR('',#37238,0.75) ;
#8742=VECTOR('',#37241,0.75) ;
#8743=VECTOR('',#37244,0.75) ;
#8744=VECTOR('',#37249,0.75) ;
#8745=VECTOR('',#37250,0.75) ;
#8746=VECTOR('',#37253,0.75) ;
#8747=VECTOR('',#37256,0.75) ;
#8748=VECTOR('',#37261,108.3) ;
#8749=VECTOR('',#37266,1.25) ;
#8750=VECTOR('',#37275,0.75) ;
#8751=VECTOR('',#37276,0.75) ;
#8752=VECTOR('',#37279,0.75) ;
#8753=VECTOR('',#37280,0.75) ;
#8754=VECTOR('',#37287,0.75) ;
#8755=VECTOR('',#37288,0.75) ;
#8756=VECTOR('',#37291,0.75) ;
#8757=VECTOR('',#37292,0.75) ;
#8758=VECTOR('',#37299,0.75) ;
#8759=VECTOR('',#37300,0.75) ;
#8760=VECTOR('',#37303,0.75) ;
#8761=VECTOR('',#37304,0.75) ;
#10873=CIRCLE('',#32775,0.25) ;
#10874=CIRCLE('',#32776,0.25) ;
#10875=CIRCLE('',#32778,23.5) ;
#10876=CIRCLE('',#32779,28.5) ;
#10877=CIRCLE('',#32780,2.4999999999) ;
#10878=CIRCLE('',#32781,28.5) ;
#10879=CIRCLE('',#32782,2.4999999999) ;
#10880=CIRCLE('',#32783,23.5) ;
#10881=CIRCLE('',#32784,2.4999999999) ;
#10882=CIRCLE('',#32785,28.5) ;
#10883=CIRCLE('',#32786,2.4999999999) ;
#10884=CIRCLE('',#32787,23.5) ;
#10885=CIRCLE('',#32788,15.5) ;
#10886=CIRCLE('',#32789,3.) ;
#10887=CIRCLE('',#32790,21.5) ;
#10888=CIRCLE('',#32791,3.) ;
#10889=CIRCLE('',#32792,1.5) ;
#10890=CIRCLE('',#32793,1.5) ;
#10891=CIRCLE('',#32794,1.5) ;
#10892=CIRCLE('',#32795,1.5) ;
#10893=CIRCLE('',#32796,1.5) ;
#10894=CIRCLE('',#32797,1.5) ;
#10895=CIRCLE('',#32798,1.5) ;
#10896=CIRCLE('',#32799,1.5) ;
#10897=CIRCLE('',#32800,1.5) ;
#10898=CIRCLE('',#32801,1.5) ;
#10899=CIRCLE('',#32802,1.5) ;
#10900=CIRCLE('',#32803,1.5) ;
#10901=CIRCLE('',#32804,1.90000000000502) ;
#10902=CIRCLE('',#32805,1.90000000000502) ;
#10903=CIRCLE('',#32806,2.) ;
#10904=CIRCLE('',#32807,2.) ;
#10905=CIRCLE('',#32808,2.) ;
#10906=CIRCLE('',#32809,2.) ;
#10907=CIRCLE('',#32810,3.) ;
#10908=CIRCLE('',#32811,21.5) ;
#10909=CIRCLE('',#32812,3.) ;
#10910=CIRCLE('',#32813,15.5) ;
#10911=CIRCLE('',#32814,3.) ;
#10912=CIRCLE('',#32815,21.5) ;
#10913=CIRCLE('',#32816,3.) ;
#10914=CIRCLE('',#32817,15.5) ;
#10915=CIRCLE('',#32818,3.) ;
#10916=CIRCLE('',#32819,21.5) ;
#10917=CIRCLE('',#32820,3.) ;
#10918=CIRCLE('',#32821,15.5) ;
#10919=CIRCLE('',#32822,23.5) ;
#10920=CIRCLE('',#32823,2.4999999999) ;
#10921=CIRCLE('',#32824,28.5) ;
#10922=CIRCLE('',#32825,2.4999999999) ;
#10923=CIRCLE('',#32827,0.25) ;
#10924=CIRCLE('',#32828,0.25) ;
#10925=CIRCLE('',#32830,0.25) ;
#10926=CIRCLE('',#32831,0.25) ;
#10927=CIRCLE('',#32833,0.5) ;
#10928=CIRCLE('',#32834,1.) ;
#10929=CIRCLE('',#32835,1.) ;
#10930=CIRCLE('',#32836,1.) ;
#10931=CIRCLE('',#32837,1.) ;
#10932=CIRCLE('',#32838,1.) ;
#10933=CIRCLE('',#32839,1.) ;
#10934=CIRCLE('',#32840,1.) ;
#10935=CIRCLE('',#32841,1.25) ;
#10936=CIRCLE('',#32842,1.25) ;
#10937=CIRCLE('',#32844,0.75) ;
#10938=CIRCLE('',#32845,0.75) ;
#10939=CIRCLE('',#32848,0.5) ;
#10940=CIRCLE('',#32849,1.) ;
#10941=CIRCLE('',#32850,1.) ;
#10942=CIRCLE('',#32851,1.) ;
#10943=CIRCLE('',#32852,1.) ;
#10944=CIRCLE('',#32853,1.) ;
#10945=CIRCLE('',#32854,1.) ;
#10946=CIRCLE('',#32855,1.) ;
#10947=CIRCLE('',#32856,1.25) ;
#10948=CIRCLE('',#32857,1.25) ;
#10949=CIRCLE('',#32859,0.75) ;
#10950=CIRCLE('',#32860,0.75) ;
#10951=CIRCLE('',#32863,1.) ;
#10952=CIRCLE('',#32864,1.) ;
#10953=CIRCLE('',#32865,1.) ;
#10954=CIRCLE('',#32866,1.) ;
#10955=CIRCLE('',#32867,1.) ;
#10956=CIRCLE('',#32868,1.) ;
#10957=CIRCLE('',#32869,1.) ;
#10958=CIRCLE('',#32870,0.5) ;
#10959=CIRCLE('',#32871,1.25) ;
#10960=CIRCLE('',#32872,1.25) ;
#10961=CIRCLE('',#32874,1.) ;
#10962=CIRCLE('',#32879,0.75) ;
#10963=CIRCLE('',#32880,0.75) ;
#10964=CIRCLE('',#32883,23.5) ;
#10965=CIRCLE('',#32884,2.4999999999) ;
#10966=CIRCLE('',#32885,28.5) ;
#10967=CIRCLE('',#32886,2.4999999999) ;
#10968=CIRCLE('',#32887,2.5) ;
#10969=CIRCLE('',#32888,2.5) ;
#10970=CIRCLE('',#32889,1.5) ;
#10971=CIRCLE('',#32890,1.5) ;
#10972=CIRCLE('',#32891,1.5) ;
#10973=CIRCLE('',#32892,1.5) ;
#10974=CIRCLE('',#32893,1.5) ;
#10975=CIRCLE('',#32894,1.5) ;
#10976=CIRCLE('',#32895,1.5) ;
#10977=CIRCLE('',#32896,1.5) ;
#10978=CIRCLE('',#32897,1.5) ;
#10979=CIRCLE('',#32898,1.5) ;
#10980=CIRCLE('',#32899,1.5) ;
#10981=CIRCLE('',#32900,1.5) ;
#10982=CIRCLE('',#32901,2.) ;
#10983=CIRCLE('',#32902,2.) ;
#10984=CIRCLE('',#32903,2.) ;
#10985=CIRCLE('',#32904,2.) ;
#10986=CIRCLE('',#32905,15.5) ;
#10987=CIRCLE('',#32906,3.) ;
#10988=CIRCLE('',#32907,21.5) ;
#10989=CIRCLE('',#32908,3.) ;
#10990=CIRCLE('',#32909,3.) ;
#10991=CIRCLE('',#32910,15.5) ;
#10992=CIRCLE('',#32911,3.) ;
#10993=CIRCLE('',#32912,21.5) ;
#10994=CIRCLE('',#32913,3.) ;
#10995=CIRCLE('',#32914,15.5) ;
#10996=CIRCLE('',#32915,3.) ;
#10997=CIRCLE('',#32916,21.5) ;
#10998=CIRCLE('',#32917,3.) ;
#10999=CIRCLE('',#32918,15.5) ;
#11000=CIRCLE('',#32919,3.) ;
#11001=CIRCLE('',#32920,21.5) ;
#11002=CIRCLE('',#32921,23.5) ;
#11003=CIRCLE('',#32922,2.4999999999) ;
#11004=CIRCLE('',#32923,28.5) ;
#11005=CIRCLE('',#32924,2.4999999999) ;
#11006=CIRCLE('',#32925,23.5) ;
#11007=CIRCLE('',#32926,2.4999999999) ;
#11008=CIRCLE('',#32927,28.5) ;
#11009=CIRCLE('',#32928,23.5) ;
#11010=CIRCLE('',#32929,2.4999999999) ;
#11011=CIRCLE('',#32930,28.5) ;
#11012=CIRCLE('',#32932,1.) ;
#11013=CIRCLE('',#32933,1.) ;
#11014=CIRCLE('',#32934,1.) ;
#11015=CIRCLE('',#32935,1.) ;
#11016=CIRCLE('',#32936,1.) ;
#11017=CIRCLE('',#32937,1.) ;
#11018=CIRCLE('',#32938,0.5) ;
#11019=CIRCLE('',#32939,1.25) ;
#11020=CIRCLE('',#32940,1.25) ;
#11021=CIRCLE('',#32942,0.5) ;
#11022=CIRCLE('',#32943,0.5) ;
#11023=CIRCLE('',#32955,0.5) ;
#11024=CIRCLE('',#32958,0.5) ;
#11025=CIRCLE('',#32962,0.5) ;
#11026=CIRCLE('',#32963,0.5) ;
#11027=CIRCLE('',#32966,0.5) ;
#11028=CIRCLE('',#32968,0.5) ;
#11029=CIRCLE('',#32970,0.75) ;
#11030=CIRCLE('',#32971,0.25) ;
#11031=CIRCLE('',#32996,0.25) ;
#11032=CIRCLE('',#32998,0.75) ;
#12667=VERTEX_POINT('',#46350) ;
#12668=VERTEX_POINT('',#46351) ;
#12669=VERTEX_POINT('',#46353) ;
#12670=VERTEX_POINT('',#46355) ;
#12671=VERTEX_POINT('',#46359) ;
#12672=VERTEX_POINT('',#46361) ;
#12673=VERTEX_POINT('',#46363) ;
#12674=VERTEX_POINT('',#46365) ;
#12675=VERTEX_POINT('',#46368) ;
#12676=VERTEX_POINT('',#46369) ;
#12677=VERTEX_POINT('',#46371) ;
#12678=VERTEX_POINT('',#46379) ;
#12679=VERTEX_POINT('',#46382) ;
#12680=VERTEX_POINT('',#46383) ;
#12681=VERTEX_POINT('',#46391) ;
#12682=VERTEX_POINT('',#46393) ;
#12683=VERTEX_POINT('',#46396) ;
#12684=VERTEX_POINT('',#46397) ;
#12685=VERTEX_POINT('',#46399) ;
#12686=VERTEX_POINT('',#46401) ;
#12687=VERTEX_POINT('',#46404) ;
#12688=VERTEX_POINT('',#46405) ;
#12689=VERTEX_POINT('',#46407) ;
#12690=VERTEX_POINT('',#46409) ;
#12691=VERTEX_POINT('',#46412) ;
#12692=VERTEX_POINT('',#46413) ;
#12693=VERTEX_POINT('',#46415) ;
#12694=VERTEX_POINT('',#46417) ;
#12695=VERTEX_POINT('',#46420) ;
#12696=VERTEX_POINT('',#46421) ;
#12697=VERTEX_POINT('',#46423) ;
#12698=VERTEX_POINT('',#46425) ;
#12699=VERTEX_POINT('',#46428) ;
#12700=VERTEX_POINT('',#46429) ;
#12701=VERTEX_POINT('',#46431) ;
#12702=VERTEX_POINT('',#46433) ;
#12703=VERTEX_POINT('',#46436) ;
#12704=VERTEX_POINT('',#46437) ;
#12705=VERTEX_POINT('',#46439) ;
#12706=VERTEX_POINT('',#46441) ;
#12707=VERTEX_POINT('',#46444) ;
#12708=VERTEX_POINT('',#46445) ;
#12709=VERTEX_POINT('',#46447) ;
#12710=VERTEX_POINT('',#46449) ;
#12711=VERTEX_POINT('',#46452) ;
#12712=VERTEX_POINT('',#46453) ;
#12713=VERTEX_POINT('',#46455) ;
#12714=VERTEX_POINT('',#46457) ;
#12715=VERTEX_POINT('',#46460) ;
#12716=VERTEX_POINT('',#46462) ;
#12717=VERTEX_POINT('',#46464) ;
#12718=VERTEX_POINT('',#46466) ;
#12719=VERTEX_POINT('',#46468) ;
#12720=VERTEX_POINT('',#46470) ;
#12721=VERTEX_POINT('',#46472) ;
#12722=VERTEX_POINT('',#46473) ;
#12723=VERTEX_POINT('',#46475) ;
#12724=VERTEX_POINT('',#46477) ;
#12725=VERTEX_POINT('',#46480) ;
#12726=VERTEX_POINT('',#46481) ;
#12727=VERTEX_POINT('',#46483) ;
#12728=VERTEX_POINT('',#46485) ;
#12729=VERTEX_POINT('',#46488) ;
#12730=VERTEX_POINT('',#46489) ;
#12731=VERTEX_POINT('',#46491) ;
#12732=VERTEX_POINT('',#46493) ;
#12733=VERTEX_POINT('',#46496) ;
#12734=VERTEX_POINT('',#46497) ;
#12735=VERTEX_POINT('',#46499) ;
#12736=VERTEX_POINT('',#46501) ;
#12737=VERTEX_POINT('',#46505) ;
#12738=VERTEX_POINT('',#46507) ;
#12739=VERTEX_POINT('',#46511) ;
#12740=VERTEX_POINT('',#46513) ;
#12741=VERTEX_POINT('',#46517) ;
#12742=VERTEX_POINT('',#46519) ;
#12743=VERTEX_POINT('',#46521) ;
#12744=VERTEX_POINT('',#46523) ;
#12745=VERTEX_POINT('',#46525) ;
#12746=VERTEX_POINT('',#46527) ;
#12747=VERTEX_POINT('',#46529) ;
#12748=VERTEX_POINT('',#46531) ;
#12749=VERTEX_POINT('',#46533) ;
#12750=VERTEX_POINT('',#46535) ;
#12751=VERTEX_POINT('',#46537) ;
#12752=VERTEX_POINT('',#46539) ;
#12753=VERTEX_POINT('',#46541) ;
#12754=VERTEX_POINT('',#46543) ;
#12755=VERTEX_POINT('',#46545) ;
#12756=VERTEX_POINT('',#46547) ;
#12757=VERTEX_POINT('',#46550) ;
#12758=VERTEX_POINT('',#46552) ;
#12759=VERTEX_POINT('',#46555) ;
#12760=VERTEX_POINT('',#46556) ;
#12761=VERTEX_POINT('',#46558) ;
#12762=VERTEX_POINT('',#46560) ;
#12763=VERTEX_POINT('',#46564) ;
#12764=VERTEX_POINT('',#46566) ;
#12765=VERTEX_POINT('',#46569) ;
#12766=VERTEX_POINT('',#46573) ;
#12767=VERTEX_POINT('',#46575) ;
#12768=VERTEX_POINT('',#46577) ;
#12769=VERTEX_POINT('',#46579) ;
#12770=VERTEX_POINT('',#46581) ;
#12771=VERTEX_POINT('',#46583) ;
#12772=VERTEX_POINT('',#46585) ;
#12773=VERTEX_POINT('',#46587) ;
#12774=VERTEX_POINT('',#46589) ;
#12775=VERTEX_POINT('',#46591) ;
#12776=VERTEX_POINT('',#46593) ;
#12777=VERTEX_POINT('',#46595) ;
#12778=VERTEX_POINT('',#46597) ;
#12779=VERTEX_POINT('',#46599) ;
#12780=VERTEX_POINT('',#46601) ;
#12781=VERTEX_POINT('',#46604) ;
#12782=VERTEX_POINT('',#46606) ;
#12783=VERTEX_POINT('',#46609) ;
#12784=VERTEX_POINT('',#46610) ;
#12785=VERTEX_POINT('',#46612) ;
#12786=VERTEX_POINT('',#46614) ;
#12787=VERTEX_POINT('',#46618) ;
#12788=VERTEX_POINT('',#46621) ;
#12789=VERTEX_POINT('',#46625) ;
#12790=VERTEX_POINT('',#46627) ;
#12791=VERTEX_POINT('',#46629) ;
#12792=VERTEX_POINT('',#46631) ;
#12793=VERTEX_POINT('',#46633) ;
#12794=VERTEX_POINT('',#46635) ;
#12795=VERTEX_POINT('',#46637) ;
#12796=VERTEX_POINT('',#46639) ;
#12797=VERTEX_POINT('',#46641) ;
#12798=VERTEX_POINT('',#46643) ;
#12799=VERTEX_POINT('',#46645) ;
#12800=VERTEX_POINT('',#46647) ;
#12801=VERTEX_POINT('',#46649) ;
#12802=VERTEX_POINT('',#46651) ;
#12803=VERTEX_POINT('',#46653) ;
#12804=VERTEX_POINT('',#46656) ;
#12805=VERTEX_POINT('',#46658) ;
#12806=VERTEX_POINT('',#46661) ;
#12807=VERTEX_POINT('',#46663) ;
#12808=VERTEX_POINT('',#46667) ;
#12809=VERTEX_POINT('',#46676) ;
#12810=VERTEX_POINT('',#46677) ;
#12811=VERTEX_POINT('',#46679) ;
#12812=VERTEX_POINT('',#46681) ;
#12813=VERTEX_POINT('',#46686) ;
#12814=VERTEX_POINT('',#46688) ;
#12815=VERTEX_POINT('',#46692) ;
#12816=VERTEX_POINT('',#46695) ;
#12817=VERTEX_POINT('',#46697) ;
#12818=VERTEX_POINT('',#46699) ;
#12819=VERTEX_POINT('',#46702) ;
#12820=VERTEX_POINT('',#46703) ;
#12821=VERTEX_POINT('',#46705) ;
#12822=VERTEX_POINT('',#46707) ;
#12823=VERTEX_POINT('',#46710) ;
#12824=VERTEX_POINT('',#46712) ;
#12825=VERTEX_POINT('',#46714) ;
#12826=VERTEX_POINT('',#46715) ;
#12827=VERTEX_POINT('',#46717) ;
#12828=VERTEX_POINT('',#46719) ;
#12829=VERTEX_POINT('',#46722) ;
#12830=VERTEX_POINT('',#46723) ;
#12831=VERTEX_POINT('',#46725) ;
#12832=VERTEX_POINT('',#46727) ;
#12833=VERTEX_POINT('',#46730) ;
#12834=VERTEX_POINT('',#46731) ;
#12835=VERTEX_POINT('',#46733) ;
#12836=VERTEX_POINT('',#46735) ;
#12837=VERTEX_POINT('',#46738) ;
#12838=VERTEX_POINT('',#46739) ;
#12839=VERTEX_POINT('',#46741) ;
#12840=VERTEX_POINT('',#46743) ;
#12841=VERTEX_POINT('',#46746) ;
#12842=VERTEX_POINT('',#46747) ;
#12843=VERTEX_POINT('',#46749) ;
#12844=VERTEX_POINT('',#46751) ;
#12845=VERTEX_POINT('',#46754) ;
#12846=VERTEX_POINT('',#46755) ;
#12847=VERTEX_POINT('',#46757) ;
#12848=VERTEX_POINT('',#46759) ;
#12849=VERTEX_POINT('',#46762) ;
#12850=VERTEX_POINT('',#46764) ;
#12851=VERTEX_POINT('',#46766) ;
#12852=VERTEX_POINT('',#46768) ;
#12853=VERTEX_POINT('',#46770) ;
#12854=VERTEX_POINT('',#46771) ;
#12855=VERTEX_POINT('',#46773) ;
#12856=VERTEX_POINT('',#46775) ;
#12857=VERTEX_POINT('',#46778) ;
#12858=VERTEX_POINT('',#46779) ;
#12859=VERTEX_POINT('',#46781) ;
#12860=VERTEX_POINT('',#46783) ;
#12861=VERTEX_POINT('',#46786) ;
#12862=VERTEX_POINT('',#46787) ;
#12863=VERTEX_POINT('',#46789) ;
#12864=VERTEX_POINT('',#46791) ;
#12865=VERTEX_POINT('',#46794) ;
#12866=VERTEX_POINT('',#46795) ;
#12867=VERTEX_POINT('',#46797) ;
#12868=VERTEX_POINT('',#46799) ;
#12869=VERTEX_POINT('',#46802) ;
#12870=VERTEX_POINT('',#46803) ;
#12871=VERTEX_POINT('',#46805) ;
#12872=VERTEX_POINT('',#46807) ;
#12873=VERTEX_POINT('',#46810) ;
#12874=VERTEX_POINT('',#46811) ;
#12875=VERTEX_POINT('',#46813) ;
#12876=VERTEX_POINT('',#46815) ;
#12877=VERTEX_POINT('',#46824) ;
#12878=VERTEX_POINT('',#46825) ;
#12879=VERTEX_POINT('',#46827) ;
#12880=VERTEX_POINT('',#46829) ;
#12881=VERTEX_POINT('',#46839) ;
#12882=VERTEX_POINT('',#46841) ;
#12883=VERTEX_POINT('',#46843) ;
#12884=VERTEX_POINT('',#46845) ;
#12885=VERTEX_POINT('',#46847) ;
#12886=VERTEX_POINT('',#46849) ;
#12887=VERTEX_POINT('',#46851) ;
#12888=VERTEX_POINT('',#46853) ;
#12889=VERTEX_POINT('',#46855) ;
#12890=VERTEX_POINT('',#46857) ;
#12891=VERTEX_POINT('',#46859) ;
#12892=VERTEX_POINT('',#46862) ;
#12893=VERTEX_POINT('',#46865) ;
#12894=VERTEX_POINT('',#46867) ;
#12895=VERTEX_POINT('',#46870) ;
#12896=VERTEX_POINT('',#46872) ;
#12897=VERTEX_POINT('',#46874) ;
#12898=VERTEX_POINT('',#46960) ;
#12899=VERTEX_POINT('',#46964) ;
#12900=VERTEX_POINT('',#46968) ;
#12901=VERTEX_POINT('',#46976) ;
#12902=VERTEX_POINT('',#46977) ;
#12903=VERTEX_POINT('',#46979) ;
#12904=VERTEX_POINT('',#46981) ;
#12905=VERTEX_POINT('',#46985) ;
#12906=VERTEX_POINT('',#46987) ;
#12907=VERTEX_POINT('',#46991) ;
#12908=VERTEX_POINT('',#46993) ;
#12909=VERTEX_POINT('',#46995) ;
#12910=VERTEX_POINT('',#46999) ;
#12911=VERTEX_POINT('',#47003) ;
#12912=VERTEX_POINT('',#47058) ;
#15596=EDGE_CURVE('',#12667,#12668,#10873,.T.) ;
#15597=EDGE_CURVE('',#12668,#12669,#6235,.T.) ;
#15598=EDGE_CURVE('',#12669,#12670,#10874,.T.) ;
#15599=EDGE_CURVE('',#12670,#12667,#6236,.T.) ;
#15600=EDGE_CURVE('',#12671,#12668,#6237,.T.) ;
#15601=EDGE_CURVE('',#12672,#12671,#6238,.T.) ;
#15602=EDGE_CURVE('',#12672,#12673,#6239,.T.) ;
#15603=EDGE_CURVE('',#12674,#12673,#6240,.T.) ;
#15604=EDGE_CURVE('',#12674,#12669,#6241,.T.) ;
#15605=EDGE_CURVE('',#12675,#12676,#10875,.F.) ;
#15606=EDGE_CURVE('',#12677,#12676,#1189,.T.) ;
#15607=EDGE_CURVE('',#12677,#12678,#10876,.T.) ;
#15608=EDGE_CURVE('',#12675,#12678,#10877,.T.) ;
#15609=EDGE_CURVE('',#12679,#12680,#1190,.T.) ;
#15610=EDGE_CURVE('',#12679,#12681,#10878,.T.) ;
#15611=EDGE_CURVE('',#12682,#12681,#10879,.T.) ;
#15612=EDGE_CURVE('',#12682,#12680,#10880,.F.) ;
#15613=EDGE_CURVE('',#12683,#12684,#10881,.T.) ;
#15614=EDGE_CURVE('',#12683,#12685,#10882,.T.) ;
#15615=EDGE_CURVE('',#12686,#12685,#10883,.T.) ;
#15616=EDGE_CURVE('',#12686,#12684,#10884,.F.) ;
#15617=EDGE_CURVE('',#12687,#12688,#10885,.F.) ;
#15618=EDGE_CURVE('',#12689,#12688,#10886,.F.) ;
#15619=EDGE_CURVE('',#12689,#12690,#10887,.T.) ;
#15620=EDGE_CURVE('',#12687,#12690,#10888,.F.) ;
#15621=EDGE_CURVE('',#12691,#12692,#6242,.F.) ;
#15622=EDGE_CURVE('',#12691,#12693,#10889,.T.) ;
#15623=EDGE_CURVE('',#12694,#12693,#6243,.F.) ;
#15624=EDGE_CURVE('',#12694,#12692,#10890,.T.) ;
#15625=EDGE_CURVE('',#12695,#12696,#6244,.F.) ;
#15626=EDGE_CURVE('',#12695,#12697,#10891,.T.) ;
#15627=EDGE_CURVE('',#12698,#12697,#6245,.F.) ;
#15628=EDGE_CURVE('',#12698,#12696,#10892,.T.) ;
#15629=EDGE_CURVE('',#12699,#12700,#6246,.F.) ;
#15630=EDGE_CURVE('',#12699,#12701,#10893,.T.) ;
#15631=EDGE_CURVE('',#12702,#12701,#6247,.F.) ;
#15632=EDGE_CURVE('',#12702,#12700,#10894,.T.) ;
#15633=EDGE_CURVE('',#12703,#12704,#6248,.F.) ;
#15634=EDGE_CURVE('',#12703,#12705,#10895,.T.) ;
#15635=EDGE_CURVE('',#12706,#12705,#6249,.F.) ;
#15636=EDGE_CURVE('',#12706,#12704,#10896,.T.) ;
#15637=EDGE_CURVE('',#12707,#12708,#6250,.F.) ;
#15638=EDGE_CURVE('',#12707,#12709,#10897,.T.) ;
#15639=EDGE_CURVE('',#12710,#12709,#6251,.F.) ;
#15640=EDGE_CURVE('',#12710,#12708,#10898,.T.) ;
#15641=EDGE_CURVE('',#12711,#12712,#6252,.F.) ;
#15642=EDGE_CURVE('',#12711,#12713,#10899,.T.) ;
#15643=EDGE_CURVE('',#12714,#12713,#6253,.F.) ;
#15644=EDGE_CURVE('',#12714,#12712,#10900,.T.) ;
#15645=EDGE_CURVE('',#12715,#12715,#10901,.T.) ;
#15646=EDGE_CURVE('',#12716,#12716,#10902,.T.) ;
#15647=EDGE_CURVE('',#12717,#12717,#10903,.T.) ;
#15648=EDGE_CURVE('',#12718,#12718,#10904,.T.) ;
#15649=EDGE_CURVE('',#12719,#12719,#10905,.T.) ;
#15650=EDGE_CURVE('',#12720,#12720,#10906,.T.) ;
#15651=EDGE_CURVE('',#12721,#12722,#10907,.F.) ;
#15652=EDGE_CURVE('',#12721,#12723,#10908,.T.) ;
#15653=EDGE_CURVE('',#12724,#12723,#10909,.F.) ;
#15654=EDGE_CURVE('',#12724,#12722,#10910,.F.) ;
#15655=EDGE_CURVE('',#12725,#12726,#10911,.F.) ;
#15656=EDGE_CURVE('',#12725,#12727,#10912,.T.) ;
#15657=EDGE_CURVE('',#12728,#12727,#10913,.F.) ;
#15658=EDGE_CURVE('',#12728,#12726,#10914,.F.) ;
#15659=EDGE_CURVE('',#12729,#12730,#10915,.F.) ;
#15660=EDGE_CURVE('',#12729,#12731,#10916,.T.) ;
#15661=EDGE_CURVE('',#12732,#12731,#10917,.F.) ;
#15662=EDGE_CURVE('',#12732,#12730,#10918,.F.) ;
#15663=EDGE_CURVE('',#12733,#12734,#10919,.F.) ;
#15664=EDGE_CURVE('',#12735,#12734,#10920,.T.) ;
#15665=EDGE_CURVE('',#12735,#12736,#10921,.T.) ;
#15666=EDGE_CURVE('',#12733,#12736,#10922,.T.) ;
#15667=EDGE_CURVE('',#12737,#12674,#10923,.T.) ;
#15668=EDGE_CURVE('',#12673,#12738,#10924,.T.) ;
#15669=EDGE_CURVE('',#12738,#12737,#6254,.T.) ;
#15670=EDGE_CURVE('',#12671,#12739,#10925,.T.) ;
#15671=EDGE_CURVE('',#12739,#12740,#6255,.T.) ;
#15672=EDGE_CURVE('',#12740,#12672,#10926,.T.) ;
#15673=EDGE_CURVE('',#12739,#12741,#6256,.F.) ;
#15674=EDGE_CURVE('',#12742,#12741,#10927,.T.) ;
#15675=EDGE_CURVE('',#12742,#12743,#6257,.F.) ;
#15676=EDGE_CURVE('',#12744,#12743,#10928,.T.) ;
#15677=EDGE_CURVE('',#12744,#12745,#6258,.F.) ;
#15678=EDGE_CURVE('',#12746,#12745,#10929,.T.) ;
#15679=EDGE_CURVE('',#12747,#12746,#6259,.T.) ;
#15680=EDGE_CURVE('',#12748,#12747,#10930,.T.) ;
#15681=EDGE_CURVE('',#12748,#12749,#6260,.F.) ;
#15682=EDGE_CURVE('',#12750,#12749,#10931,.T.) ;
#15683=EDGE_CURVE('',#12750,#12751,#6261,.F.) ;
#15684=EDGE_CURVE('',#12752,#12751,#10932,.T.) ;
#15685=EDGE_CURVE('',#12752,#12753,#6262,.F.) ;
#15686=EDGE_CURVE('',#12754,#12753,#10933,.T.) ;
#15687=EDGE_CURVE('',#12755,#12754,#6263,.T.) ;
#15688=EDGE_CURVE('',#12756,#12755,#10934,.T.) ;
#15689=EDGE_CURVE('',#12756,#12740,#6264,.F.) ;
#15690=EDGE_CURVE('',#12757,#12757,#10935,.F.) ;
#15691=EDGE_CURVE('',#12758,#12758,#10936,.F.) ;
#15692=EDGE_CURVE('',#12759,#12760,#10937,.T.) ;
#15693=EDGE_CURVE('',#12760,#12761,#6265,.T.) ;
#15694=EDGE_CURVE('',#12761,#12762,#10938,.T.) ;
#15695=EDGE_CURVE('',#12762,#12759,#6266,.T.) ;
#15696=EDGE_CURVE('',#12763,#12759,#6267,.T.) ;
#15697=EDGE_CURVE('',#12764,#12763,#6268,.T.) ;
#15698=EDGE_CURVE('',#12670,#12764,#6269,.T.) ;
#15699=EDGE_CURVE('',#12765,#12674,#6270,.F.) ;
#15700=EDGE_CURVE('',#12760,#12765,#6271,.T.) ;
#15701=EDGE_CURVE('',#12762,#12766,#6272,.T.) ;
#15702=EDGE_CURVE('',#12767,#12766,#10939,.T.) ;
#15703=EDGE_CURVE('',#12768,#12767,#6273,.T.) ;
#15704=EDGE_CURVE('',#12769,#12768,#10940,.T.) ;
#15705=EDGE_CURVE('',#12770,#12769,#6274,.T.) ;
#15706=EDGE_CURVE('',#12771,#12770,#10941,.T.) ;
#15707=EDGE_CURVE('',#12772,#12771,#6275,.F.) ;
#15708=EDGE_CURVE('',#12773,#12772,#10942,.T.) ;
#15709=EDGE_CURVE('',#12774,#12773,#6276,.T.) ;
#15710=EDGE_CURVE('',#12775,#12774,#10943,.T.) ;
#15711=EDGE_CURVE('',#12776,#12775,#6277,.T.) ;
#15712=EDGE_CURVE('',#12777,#12776,#10944,.T.) ;
#15713=EDGE_CURVE('',#12777,#12778,#6278,.T.) ;
#15714=EDGE_CURVE('',#12779,#12778,#10945,.T.) ;
#15715=EDGE_CURVE('',#12780,#12779,#6279,.T.) ;
#15716=EDGE_CURVE('',#12763,#12780,#10946,.T.) ;
#15717=EDGE_CURVE('',#12781,#12781,#10947,.T.) ;
#15718=EDGE_CURVE('',#12782,#12782,#10948,.T.) ;
#15719=EDGE_CURVE('',#12783,#12784,#10949,.T.) ;
#15720=EDGE_CURVE('',#12784,#12785,#6280,.T.) ;
#15721=EDGE_CURVE('',#12785,#12786,#10950,.T.) ;
#15722=EDGE_CURVE('',#12786,#12783,#6281,.T.) ;
#15723=EDGE_CURVE('',#12787,#12783,#6282,.T.) ;
#15724=EDGE_CURVE('',#12741,#12787,#6283,.T.) ;
#15725=EDGE_CURVE('',#12788,#12671,#6284,.T.) ;
#15726=EDGE_CURVE('',#12784,#12788,#6285,.T.) ;
#15727=EDGE_CURVE('',#12789,#12786,#6286,.T.) ;
#15728=EDGE_CURVE('',#12790,#12789,#10951,.T.) ;
#15729=EDGE_CURVE('',#12791,#12790,#6287,.T.) ;
#15730=EDGE_CURVE('',#12792,#12791,#10952,.T.) ;
#15731=EDGE_CURVE('',#12792,#12793,#6288,.T.) ;
#15732=EDGE_CURVE('',#12794,#12793,#10953,.T.) ;
#15733=EDGE_CURVE('',#12794,#12795,#6289,.T.) ;
#15734=EDGE_CURVE('',#12796,#12795,#10954,.T.) ;
#15735=EDGE_CURVE('',#12796,#12797,#6290,.T.) ;
#15736=EDGE_CURVE('',#12798,#12797,#10955,.T.) ;
#15737=EDGE_CURVE('',#12799,#12798,#6291,.T.) ;
#15738=EDGE_CURVE('',#12800,#12799,#10956,.T.) ;
#15739=EDGE_CURVE('',#12800,#12801,#6292,.T.) ;
#15740=EDGE_CURVE('',#12802,#12801,#10957,.T.) ;
#15741=EDGE_CURVE('',#12802,#12803,#6293,.T.) ;
#15742=EDGE_CURVE('',#12787,#12803,#10958,.T.) ;
#15743=EDGE_CURVE('',#12804,#12804,#10959,.T.) ;
#15744=EDGE_CURVE('',#12805,#12805,#10960,.T.) ;
#15745=EDGE_CURVE('',#12768,#12806,#6294,.T.) ;
#15746=EDGE_CURVE('',#12806,#12807,#10961,.T.) ;
#15747=EDGE_CURVE('',#12807,#12769,#6295,.T.) ;
#15748=EDGE_CURVE('',#12808,#12767,#6296,.T.) ;
#15749=EDGE_CURVE('',#12806,#12808,#6297,.T.) ;
#15750=EDGE_CURVE('',#12743,#12802,#6298,.T.) ;
#15751=EDGE_CURVE('',#12801,#12744,#6299,.T.) ;
#15752=EDGE_CURVE('',#12803,#12742,#6300,.T.) ;
#15753=EDGE_CURVE('',#12809,#12810,#10962,.T.) ;
#15754=EDGE_CURVE('',#12810,#12811,#6301,.T.) ;
#15755=EDGE_CURVE('',#12811,#12812,#10963,.T.) ;
#15756=EDGE_CURVE('',#12812,#12809,#6302,.T.) ;
#15757=EDGE_CURVE('',#12811,#12765,#6303,.F.) ;
#15758=EDGE_CURVE('',#12813,#12737,#6304,.F.) ;
#15759=EDGE_CURVE('',#12814,#12813,#6305,.T.) ;
#15760=EDGE_CURVE('',#12812,#12814,#6306,.F.) ;
#15761=EDGE_CURVE('',#12815,#12810,#6307,.F.) ;
#15762=EDGE_CURVE('',#12785,#12815,#6308,.T.) ;
#15763=EDGE_CURVE('',#12816,#12788,#6309,.T.) ;
#15764=EDGE_CURVE('',#12817,#12816,#6310,.T.) ;
#15765=EDGE_CURVE('',#12818,#12817,#6311,.T.) ;
#15766=EDGE_CURVE('',#12761,#12818,#6312,.T.) ;
#15767=EDGE_CURVE('',#12819,#12820,#10964,.T.) ;
#15768=EDGE_CURVE('',#12821,#12820,#10965,.T.) ;
#15769=EDGE_CURVE('',#12822,#12821,#10966,.T.) ;
#15770=EDGE_CURVE('',#12819,#12822,#10967,.T.) ;
#15771=EDGE_CURVE('',#12823,#12823,#10968,.T.) ;
#15772=EDGE_CURVE('',#12824,#12824,#10969,.T.) ;
#15773=EDGE_CURVE('',#12825,#12826,#10970,.T.) ;
#15774=EDGE_CURVE('',#12827,#12826,#6313,.T.) ;
#15775=EDGE_CURVE('',#12827,#12828,#10971,.T.) ;
#15776=EDGE_CURVE('',#12825,#12828,#6314,.T.) ;
#15777=EDGE_CURVE('',#12829,#12830,#10972,.T.) ;
#15778=EDGE_CURVE('',#12831,#12830,#6315,.T.) ;
#15779=EDGE_CURVE('',#12831,#12832,#10973,.T.) ;
#15780=EDGE_CURVE('',#12829,#12832,#6316,.T.) ;
#15781=EDGE_CURVE('',#12833,#12834,#10974,.T.) ;
#15782=EDGE_CURVE('',#12835,#12834,#6317,.T.) ;
#15783=EDGE_CURVE('',#12835,#12836,#10975,.T.) ;
#15784=EDGE_CURVE('',#12833,#12836,#6318,.T.) ;
#15785=EDGE_CURVE('',#12837,#12838,#10976,.T.) ;
#15786=EDGE_CURVE('',#12839,#12838,#6319,.T.) ;
#15787=EDGE_CURVE('',#12839,#12840,#10977,.T.) ;
#15788=EDGE_CURVE('',#12837,#12840,#6320,.T.) ;
#15789=EDGE_CURVE('',#12841,#12842,#10978,.T.) ;
#15790=EDGE_CURVE('',#12843,#12842,#6321,.T.) ;
#15791=EDGE_CURVE('',#12843,#12844,#10979,.T.) ;
#15792=EDGE_CURVE('',#12841,#12844,#6322,.T.) ;
#15793=EDGE_CURVE('',#12845,#12846,#10980,.T.) ;
#15794=EDGE_CURVE('',#12847,#12846,#6323,.T.) ;
#15795=EDGE_CURVE('',#12847,#12848,#10981,.T.) ;
#15796=EDGE_CURVE('',#12845,#12848,#6324,.T.) ;
#15797=EDGE_CURVE('',#12849,#12849,#10982,.T.) ;
#15798=EDGE_CURVE('',#12850,#12850,#10983,.T.) ;
#15799=EDGE_CURVE('',#12851,#12851,#10984,.T.) ;
#15800=EDGE_CURVE('',#12852,#12852,#10985,.T.) ;
#15801=EDGE_CURVE('',#12853,#12854,#10986,.T.) ;
#15802=EDGE_CURVE('',#12855,#12854,#10987,.T.) ;
#15803=EDGE_CURVE('',#12855,#12856,#10988,.T.) ;
#15804=EDGE_CURVE('',#12853,#12856,#10989,.T.) ;
#15805=EDGE_CURVE('',#12857,#12858,#10990,.T.) ;
#15806=EDGE_CURVE('',#12857,#12859,#10991,.T.) ;
#15807=EDGE_CURVE('',#12860,#12859,#10992,.T.) ;
#15808=EDGE_CURVE('',#12860,#12858,#10993,.T.) ;
#15809=EDGE_CURVE('',#12861,#12862,#10994,.T.) ;
#15810=EDGE_CURVE('',#12861,#12863,#10995,.T.) ;
#15811=EDGE_CURVE('',#12864,#12863,#10996,.T.) ;
#15812=EDGE_CURVE('',#12864,#12862,#10997,.T.) ;
#15813=EDGE_CURVE('',#12865,#12866,#10998,.T.) ;
#15814=EDGE_CURVE('',#12865,#12867,#10999,.T.) ;
#15815=EDGE_CURVE('',#12868,#12867,#11000,.T.) ;
#15816=EDGE_CURVE('',#12868,#12866,#11001,.T.) ;
#15817=EDGE_CURVE('',#12869,#12870,#11002,.T.) ;
#15818=EDGE_CURVE('',#12871,#12870,#11003,.T.) ;
#15819=EDGE_CURVE('',#12872,#12871,#11004,.T.) ;
#15820=EDGE_CURVE('',#12869,#12872,#11005,.T.) ;
#15821=EDGE_CURVE('',#12873,#12874,#11006,.T.) ;
#15822=EDGE_CURVE('',#12875,#12874,#11007,.T.) ;
#15823=EDGE_CURVE('',#12876,#12875,#11008,.T.) ;
#15824=EDGE_CURVE('',#12873,#12876,#1191,.T.) ;
#15825=EDGE_CURVE('',#12877,#12878,#11009,.T.) ;
#15826=EDGE_CURVE('',#12879,#12878,#11010,.T.) ;
#15827=EDGE_CURVE('',#12880,#12879,#11011,.T.) ;
#15828=EDGE_CURVE('',#12877,#12880,#1192,.T.) ;
#15829=EDGE_CURVE('',#12881,#12764,#11012,.T.) ;
#15830=EDGE_CURVE('',#12882,#12881,#6325,.T.) ;
#15831=EDGE_CURVE('',#12883,#12882,#11013,.T.) ;
#15832=EDGE_CURVE('',#12883,#12884,#6326,.F.) ;
#15833=EDGE_CURVE('',#12885,#12884,#11014,.T.) ;
#15834=EDGE_CURVE('',#12885,#12886,#6327,.T.) ;
#15835=EDGE_CURVE('',#12887,#12886,#11015,.T.) ;
#15836=EDGE_CURVE('',#12887,#12888,#6328,.F.) ;
#15837=EDGE_CURVE('',#12889,#12888,#11016,.T.) ;
#15838=EDGE_CURVE('',#12889,#12890,#6329,.F.) ;
#15839=EDGE_CURVE('',#12891,#12890,#11017,.T.) ;
#15840=EDGE_CURVE('',#12891,#12807,#6330,.F.) ;
#15841=EDGE_CURVE('',#12892,#12808,#11018,.T.) ;
#15842=EDGE_CURVE('',#12892,#12667,#6331,.T.) ;
#15843=EDGE_CURVE('',#12893,#12893,#11019,.F.) ;
#15844=EDGE_CURVE('',#12894,#12894,#11020,.T.) ;
#15845=EDGE_CURVE('',#12738,#12895,#6332,.F.) ;
#15846=EDGE_CURVE('',#12896,#12895,#11021,.T.) ;
#15847=EDGE_CURVE('',#12896,#12897,#6333,.F.) ;
#15848=EDGE_CURVE('',#12813,#12897,#11022,.T.) ;
#15849=EDGE_CURVE('',#12736,#12821,#6334,.T.) ;
#15850=EDGE_CURVE('',#12733,#12820,#6335,.T.) ;
#15851=EDGE_CURVE('',#12822,#12735,#6336,.T.) ;
#15852=EDGE_CURVE('',#12872,#12683,#6337,.T.) ;
#15853=EDGE_CURVE('',#12684,#12869,#6338,.T.) ;
#15854=EDGE_CURVE('',#12685,#12871,#6339,.T.) ;
#15855=EDGE_CURVE('',#12686,#12870,#6340,.T.) ;
#15856=EDGE_CURVE('',#12876,#12679,#6341,.T.) ;
#15857=EDGE_CURVE('',#12680,#12873,#6342,.T.) ;
#15858=EDGE_CURVE('',#12681,#12875,#6343,.T.) ;
#15859=EDGE_CURVE('',#12682,#12874,#6344,.T.) ;
#15860=EDGE_CURVE('',#12880,#12677,#6345,.T.) ;
#15861=EDGE_CURVE('',#12676,#12877,#6346,.T.) ;
#15862=EDGE_CURVE('',#12678,#12879,#6347,.T.) ;
#15863=EDGE_CURVE('',#12675,#12878,#6348,.T.) ;
#15864=EDGE_CURVE('',#12734,#12819,#6349,.T.) ;
#15865=EDGE_CURVE('',#12897,#12898,#6350,.T.) ;
#15866=EDGE_CURVE('',#12898,#12814,#11023,.T.) ;
#15867=EDGE_CURVE('',#12899,#12896,#6351,.T.) ;
#15868=EDGE_CURVE('',#12898,#12899,#6352,.F.) ;
#15869=EDGE_CURVE('',#12895,#12900,#6353,.T.) ;
#15870=EDGE_CURVE('',#12900,#12899,#11024,.T.) ;
#15871=EDGE_CURVE('',#12809,#12900,#6354,.T.) ;
#15872=EDGE_CURVE('',#12815,#12673,#6355,.T.) ;
#15873=EDGE_CURVE('',#12901,#12902,#11025,.T.) ;
#15874=EDGE_CURVE('',#12902,#12903,#6356,.T.) ;
#15875=EDGE_CURVE('',#12903,#12904,#11026,.T.) ;
#15876=EDGE_CURVE('',#12904,#12901,#6357,.T.) ;
#15877=EDGE_CURVE('',#12902,#12905,#6358,.F.) ;
#15878=EDGE_CURVE('',#12906,#12905,#6359,.T.) ;
#15879=EDGE_CURVE('',#12906,#12903,#6360,.T.) ;
#15880=EDGE_CURVE('',#12901,#12907,#6361,.T.) ;
#15881=EDGE_CURVE('',#12908,#12907,#6362,.T.) ;
#15882=EDGE_CURVE('',#12908,#12909,#6363,.T.) ;
#15883=EDGE_CURVE('',#12905,#12909,#11027,.T.) ;
#15884=EDGE_CURVE('',#12910,#12906,#11028,.T.) ;
#15885=EDGE_CURVE('',#12909,#12910,#6364,.T.) ;
#15886=EDGE_CURVE('',#12817,#12911,#11029,.T.) ;
#15887=EDGE_CURVE('',#12911,#12910,#6365,.T.) ;
#15888=EDGE_CURVE('',#12668,#12908,#11030,.T.) ;
#15889=EDGE_CURVE('',#12818,#12668,#6366,.F.) ;
#15890=EDGE_CURVE('',#12766,#12892,#6367,.T.) ;
#15891=EDGE_CURVE('',#12799,#12746,#6368,.T.) ;
#15892=EDGE_CURVE('',#12745,#12800,#6369,.T.) ;
#15893=EDGE_CURVE('',#12747,#12798,#6370,.T.) ;
#15894=EDGE_CURVE('',#12749,#12796,#6371,.T.) ;
#15895=EDGE_CURVE('',#12795,#12750,#6372,.T.) ;
#15896=EDGE_CURVE('',#12797,#12748,#6373,.T.) ;
#15897=EDGE_CURVE('',#12791,#12754,#6374,.T.) ;
#15898=EDGE_CURVE('',#12753,#12792,#6375,.T.) ;
#15899=EDGE_CURVE('',#12755,#12790,#6376,.T.) ;
#15900=EDGE_CURVE('',#12751,#12794,#6377,.T.) ;
#15901=EDGE_CURVE('',#12793,#12752,#6378,.T.) ;
#15902=EDGE_CURVE('',#12789,#12756,#6379,.T.) ;
#15903=EDGE_CURVE('',#12884,#12777,#6380,.T.) ;
#15904=EDGE_CURVE('',#12776,#12885,#6381,.T.) ;
#15905=EDGE_CURVE('',#12778,#12883,#6382,.T.) ;
#15906=EDGE_CURVE('',#12882,#12779,#6383,.T.) ;
#15907=EDGE_CURVE('',#12780,#12881,#6384,.T.) ;
#15908=EDGE_CURVE('',#12774,#12887,#6385,.T.) ;
#15909=EDGE_CURVE('',#12886,#12775,#6386,.T.) ;
#15910=EDGE_CURVE('',#12888,#12773,#6387,.T.) ;
#15911=EDGE_CURVE('',#12772,#12889,#6388,.T.) ;
#15912=EDGE_CURVE('',#12770,#12891,#6389,.T.) ;
#15913=EDGE_CURVE('',#12890,#12771,#6390,.T.) ;
#15914=EDGE_CURVE('',#12907,#12671,#11031,.T.) ;
#15915=EDGE_CURVE('',#12912,#12904,#6391,.T.) ;
#15916=EDGE_CURVE('',#12912,#12816,#11032,.T.) ;
#15917=EDGE_CURVE('',#12758,#12805,#6392,.T.) ;
#15918=EDGE_CURVE('',#12757,#12804,#6393,.T.) ;
#15919=EDGE_CURVE('',#12782,#12894,#6394,.T.) ;
#15920=EDGE_CURVE('',#12853,#12688,#6395,.T.) ;
#15921=EDGE_CURVE('',#12856,#12689,#6396,.T.) ;
#15922=EDGE_CURVE('',#12855,#12690,#6397,.T.) ;
#15923=EDGE_CURVE('',#12687,#12854,#6398,.T.) ;
#15924=EDGE_CURVE('',#12716,#12823,#6399,.T.) ;
#15925=EDGE_CURVE('',#12715,#12824,#6400,.T.) ;
#15926=EDGE_CURVE('',#12717,#12852,#6401,.T.) ;
#15927=EDGE_CURVE('',#12718,#12851,#6402,.T.) ;
#15928=EDGE_CURVE('',#12719,#12850,#6403,.T.) ;
#15929=EDGE_CURVE('',#12720,#12849,#6404,.T.) ;
#15930=EDGE_CURVE('',#12847,#12713,#6405,.T.) ;
#15931=EDGE_CURVE('',#12711,#12848,#6406,.T.) ;
#15932=EDGE_CURVE('',#12714,#12846,#6407,.T.) ;
#15933=EDGE_CURVE('',#12845,#12712,#6408,.T.) ;
#15934=EDGE_CURVE('',#12843,#12709,#6409,.T.) ;
#15935=EDGE_CURVE('',#12707,#12844,#6410,.T.) ;
#15936=EDGE_CURVE('',#12710,#12842,#6411,.T.) ;
#15937=EDGE_CURVE('',#12841,#12708,#6412,.T.) ;
#15938=EDGE_CURVE('',#12839,#12705,#6413,.T.) ;
#15939=EDGE_CURVE('',#12703,#12840,#6414,.T.) ;
#15940=EDGE_CURVE('',#12706,#12838,#6415,.T.) ;
#15941=EDGE_CURVE('',#12837,#12704,#6416,.T.) ;
#15942=EDGE_CURVE('',#12835,#12701,#6417,.T.) ;
#15943=EDGE_CURVE('',#12699,#12836,#6418,.T.) ;
#15944=EDGE_CURVE('',#12702,#12834,#6419,.T.) ;
#15945=EDGE_CURVE('',#12833,#12700,#6420,.T.) ;
#15946=EDGE_CURVE('',#12831,#12697,#6421,.T.) ;
#15947=EDGE_CURVE('',#12695,#12832,#6422,.T.) ;
#15948=EDGE_CURVE('',#12698,#12830,#6423,.T.) ;
#15949=EDGE_CURVE('',#12829,#12696,#6424,.T.) ;
#15950=EDGE_CURVE('',#12827,#12693,#6425,.T.) ;
#15951=EDGE_CURVE('',#12691,#12828,#6426,.T.) ;
#15952=EDGE_CURVE('',#12694,#12826,#6427,.T.) ;
#15953=EDGE_CURVE('',#12825,#12692,#6428,.T.) ;
#15954=EDGE_CURVE('',#12912,#12911,#6429,.T.) ;
#15955=EDGE_CURVE('',#12781,#12893,#6430,.T.) ;
#15956=EDGE_CURVE('',#12857,#12722,#6431,.T.) ;
#15957=EDGE_CURVE('',#12858,#12721,#6432,.T.) ;
#15958=EDGE_CURVE('',#12860,#12723,#6433,.T.) ;
#15959=EDGE_CURVE('',#12724,#12859,#6434,.T.) ;
#15960=EDGE_CURVE('',#12861,#12726,#6435,.T.) ;
#15961=EDGE_CURVE('',#12862,#12725,#6436,.T.) ;
#15962=EDGE_CURVE('',#12864,#12727,#6437,.T.) ;
#15963=EDGE_CURVE('',#12728,#12863,#6438,.T.) ;
#15964=EDGE_CURVE('',#12865,#12730,#6439,.T.) ;
#15965=EDGE_CURVE('',#12866,#12729,#6440,.T.) ;
#15966=EDGE_CURVE('',#12868,#12731,#6441,.T.) ;
#15967=EDGE_CURVE('',#12732,#12867,#6442,.T.) ;
#20380=ORIENTED_EDGE('',*,*,#15596,.T.) ;
#20381=ORIENTED_EDGE('',*,*,#15597,.T.) ;
#20382=ORIENTED_EDGE('',*,*,#15598,.T.) ;
#20383=ORIENTED_EDGE('',*,*,#15599,.T.) ;
#20384=ORIENTED_EDGE('',*,*,#15597,.F.) ;
#20385=ORIENTED_EDGE('',*,*,#15600,.F.) ;
#20386=ORIENTED_EDGE('',*,*,#15601,.F.) ;
#20387=ORIENTED_EDGE('',*,*,#15602,.T.) ;
#20388=ORIENTED_EDGE('',*,*,#15603,.F.) ;
#20389=ORIENTED_EDGE('',*,*,#15604,.T.) ;
#20390=ORIENTED_EDGE('',*,*,#15605,.T.) ;
#20391=ORIENTED_EDGE('',*,*,#15606,.F.) ;
#20392=ORIENTED_EDGE('',*,*,#15607,.T.) ;
#20393=ORIENTED_EDGE('',*,*,#15608,.F.) ;
#20394=ORIENTED_EDGE('',*,*,#15609,.F.) ;
#20395=ORIENTED_EDGE('',*,*,#15610,.T.) ;
#20396=ORIENTED_EDGE('',*,*,#15611,.F.) ;
#20397=ORIENTED_EDGE('',*,*,#15612,.T.) ;
#20398=ORIENTED_EDGE('',*,*,#15613,.F.) ;
#20399=ORIENTED_EDGE('',*,*,#15614,.T.) ;
#20400=ORIENTED_EDGE('',*,*,#15615,.F.) ;
#20401=ORIENTED_EDGE('',*,*,#15616,.T.) ;
#20402=ORIENTED_EDGE('',*,*,#15617,.T.) ;
#20403=ORIENTED_EDGE('',*,*,#15618,.F.) ;
#20404=ORIENTED_EDGE('',*,*,#15619,.T.) ;
#20405=ORIENTED_EDGE('',*,*,#15620,.F.) ;
#20406=ORIENTED_EDGE('',*,*,#15621,.F.) ;
#20407=ORIENTED_EDGE('',*,*,#15622,.T.) ;
#20408=ORIENTED_EDGE('',*,*,#15623,.F.) ;
#20409=ORIENTED_EDGE('',*,*,#15624,.T.) ;
#20410=ORIENTED_EDGE('',*,*,#15625,.F.) ;
#20411=ORIENTED_EDGE('',*,*,#15626,.T.) ;
#20412=ORIENTED_EDGE('',*,*,#15627,.F.) ;
#20413=ORIENTED_EDGE('',*,*,#15628,.T.) ;
#20414=ORIENTED_EDGE('',*,*,#15629,.F.) ;
#20415=ORIENTED_EDGE('',*,*,#15630,.T.) ;
#20416=ORIENTED_EDGE('',*,*,#15631,.F.) ;
#20417=ORIENTED_EDGE('',*,*,#15632,.T.) ;
#20418=ORIENTED_EDGE('',*,*,#15633,.F.) ;
#20419=ORIENTED_EDGE('',*,*,#15634,.T.) ;
#20420=ORIENTED_EDGE('',*,*,#15635,.F.) ;
#20421=ORIENTED_EDGE('',*,*,#15636,.T.) ;
#20422=ORIENTED_EDGE('',*,*,#15637,.F.) ;
#20423=ORIENTED_EDGE('',*,*,#15638,.T.) ;
#20424=ORIENTED_EDGE('',*,*,#15639,.F.) ;
#20425=ORIENTED_EDGE('',*,*,#15640,.T.) ;
#20426=ORIENTED_EDGE('',*,*,#15641,.F.) ;
#20427=ORIENTED_EDGE('',*,*,#15642,.T.) ;
#20428=ORIENTED_EDGE('',*,*,#15643,.F.) ;
#20429=ORIENTED_EDGE('',*,*,#15644,.T.) ;
#20430=ORIENTED_EDGE('',*,*,#15645,.T.) ;
#20431=ORIENTED_EDGE('',*,*,#15646,.T.) ;
#20432=ORIENTED_EDGE('',*,*,#15647,.T.) ;
#20433=ORIENTED_EDGE('',*,*,#15648,.T.) ;
#20434=ORIENTED_EDGE('',*,*,#15649,.T.) ;
#20435=ORIENTED_EDGE('',*,*,#15650,.T.) ;
#20436=ORIENTED_EDGE('',*,*,#15651,.F.) ;
#20437=ORIENTED_EDGE('',*,*,#15652,.T.) ;
#20438=ORIENTED_EDGE('',*,*,#15653,.F.) ;
#20439=ORIENTED_EDGE('',*,*,#15654,.T.) ;
#20440=ORIENTED_EDGE('',*,*,#15655,.F.) ;
#20441=ORIENTED_EDGE('',*,*,#15656,.T.) ;
#20442=ORIENTED_EDGE('',*,*,#15657,.F.) ;
#20443=ORIENTED_EDGE('',*,*,#15658,.T.) ;
#20444=ORIENTED_EDGE('',*,*,#15659,.F.) ;
#20445=ORIENTED_EDGE('',*,*,#15660,.T.) ;
#20446=ORIENTED_EDGE('',*,*,#15661,.F.) ;
#20447=ORIENTED_EDGE('',*,*,#15662,.T.) ;
#20448=ORIENTED_EDGE('',*,*,#15663,.T.) ;
#20449=ORIENTED_EDGE('',*,*,#15664,.F.) ;
#20450=ORIENTED_EDGE('',*,*,#15665,.T.) ;
#20451=ORIENTED_EDGE('',*,*,#15666,.F.) ;
#20452=ORIENTED_EDGE('',*,*,#15667,.T.) ;
#20453=ORIENTED_EDGE('',*,*,#15603,.T.) ;
#20454=ORIENTED_EDGE('',*,*,#15668,.T.) ;
#20455=ORIENTED_EDGE('',*,*,#15669,.T.) ;
#20456=ORIENTED_EDGE('',*,*,#15670,.T.) ;
#20457=ORIENTED_EDGE('',*,*,#15671,.T.) ;
#20458=ORIENTED_EDGE('',*,*,#15672,.T.) ;
#20459=ORIENTED_EDGE('',*,*,#15601,.T.) ;
#20460=ORIENTED_EDGE('',*,*,#15671,.F.) ;
#20461=ORIENTED_EDGE('',*,*,#15673,.T.) ;
#20462=ORIENTED_EDGE('',*,*,#15674,.F.) ;
#20463=ORIENTED_EDGE('',*,*,#15675,.T.) ;
#20464=ORIENTED_EDGE('',*,*,#15676,.F.) ;
#20465=ORIENTED_EDGE('',*,*,#15677,.T.) ;
#20466=ORIENTED_EDGE('',*,*,#15678,.F.) ;
#20467=ORIENTED_EDGE('',*,*,#15679,.F.) ;
#20468=ORIENTED_EDGE('',*,*,#15680,.F.) ;
#20469=ORIENTED_EDGE('',*,*,#15681,.T.) ;
#20470=ORIENTED_EDGE('',*,*,#15682,.F.) ;
#20471=ORIENTED_EDGE('',*,*,#15683,.T.) ;
#20472=ORIENTED_EDGE('',*,*,#15684,.F.) ;
#20473=ORIENTED_EDGE('',*,*,#15685,.T.) ;
#20474=ORIENTED_EDGE('',*,*,#15686,.F.) ;
#20475=ORIENTED_EDGE('',*,*,#15687,.F.) ;
#20476=ORIENTED_EDGE('',*,*,#15688,.F.) ;
#20477=ORIENTED_EDGE('',*,*,#15689,.T.) ;
#20478=ORIENTED_EDGE('',*,*,#15690,.T.) ;
#20479=ORIENTED_EDGE('',*,*,#15691,.T.) ;
#20480=ORIENTED_EDGE('',*,*,#15692,.T.) ;
#20481=ORIENTED_EDGE('',*,*,#15693,.T.) ;
#20482=ORIENTED_EDGE('',*,*,#15694,.T.) ;
#20483=ORIENTED_EDGE('',*,*,#15695,.T.) ;
#20484=ORIENTED_EDGE('',*,*,#15692,.F.) ;
#20485=ORIENTED_EDGE('',*,*,#15696,.F.) ;
#20486=ORIENTED_EDGE('',*,*,#15697,.F.) ;
#20487=ORIENTED_EDGE('',*,*,#15698,.F.) ;
#20488=ORIENTED_EDGE('',*,*,#15598,.F.) ;
#20489=ORIENTED_EDGE('',*,*,#15604,.F.) ;
#20490=ORIENTED_EDGE('',*,*,#15699,.F.) ;
#20491=ORIENTED_EDGE('',*,*,#15700,.F.) ;
#20492=ORIENTED_EDGE('',*,*,#15695,.F.) ;
#20493=ORIENTED_EDGE('',*,*,#15701,.T.) ;
#20494=ORIENTED_EDGE('',*,*,#15702,.F.) ;
#20495=ORIENTED_EDGE('',*,*,#15703,.F.) ;
#20496=ORIENTED_EDGE('',*,*,#15704,.F.) ;
#20497=ORIENTED_EDGE('',*,*,#15705,.F.) ;
#20498=ORIENTED_EDGE('',*,*,#15706,.F.) ;
#20499=ORIENTED_EDGE('',*,*,#15707,.F.) ;
#20500=ORIENTED_EDGE('',*,*,#15708,.F.) ;
#20501=ORIENTED_EDGE('',*,*,#15709,.F.) ;
#20502=ORIENTED_EDGE('',*,*,#15710,.F.) ;
#20503=ORIENTED_EDGE('',*,*,#15711,.F.) ;
#20504=ORIENTED_EDGE('',*,*,#15712,.F.) ;
#20505=ORIENTED_EDGE('',*,*,#15713,.T.) ;
#20506=ORIENTED_EDGE('',*,*,#15714,.F.) ;
#20507=ORIENTED_EDGE('',*,*,#15715,.F.) ;
#20508=ORIENTED_EDGE('',*,*,#15716,.F.) ;
#20509=ORIENTED_EDGE('',*,*,#15696,.T.) ;
#20510=ORIENTED_EDGE('',*,*,#15717,.F.) ;
#20511=ORIENTED_EDGE('',*,*,#15718,.T.) ;
#20512=ORIENTED_EDGE('',*,*,#15719,.T.) ;
#20513=ORIENTED_EDGE('',*,*,#15720,.T.) ;
#20514=ORIENTED_EDGE('',*,*,#15721,.T.) ;
#20515=ORIENTED_EDGE('',*,*,#15722,.T.) ;
#20516=ORIENTED_EDGE('',*,*,#15719,.F.) ;
#20517=ORIENTED_EDGE('',*,*,#15723,.F.) ;
#20518=ORIENTED_EDGE('',*,*,#15724,.F.) ;
#20519=ORIENTED_EDGE('',*,*,#15673,.F.) ;
#20520=ORIENTED_EDGE('',*,*,#15670,.F.) ;
#20521=ORIENTED_EDGE('',*,*,#15725,.F.) ;
#20522=ORIENTED_EDGE('',*,*,#15726,.F.) ;
#20523=ORIENTED_EDGE('',*,*,#15722,.F.) ;
#20524=ORIENTED_EDGE('',*,*,#15727,.F.) ;
#20525=ORIENTED_EDGE('',*,*,#15728,.F.) ;
#20526=ORIENTED_EDGE('',*,*,#15729,.F.) ;
#20527=ORIENTED_EDGE('',*,*,#15730,.F.) ;
#20528=ORIENTED_EDGE('',*,*,#15731,.T.) ;
#20529=ORIENTED_EDGE('',*,*,#15732,.F.) ;
#20530=ORIENTED_EDGE('',*,*,#15733,.T.) ;
#20531=ORIENTED_EDGE('',*,*,#15734,.F.) ;
#20532=ORIENTED_EDGE('',*,*,#15735,.T.) ;
#20533=ORIENTED_EDGE('',*,*,#15736,.F.) ;
#20534=ORIENTED_EDGE('',*,*,#15737,.F.) ;
#20535=ORIENTED_EDGE('',*,*,#15738,.F.) ;
#20536=ORIENTED_EDGE('',*,*,#15739,.T.) ;
#20537=ORIENTED_EDGE('',*,*,#15740,.F.) ;
#20538=ORIENTED_EDGE('',*,*,#15741,.T.) ;
#20539=ORIENTED_EDGE('',*,*,#15742,.F.) ;
#20540=ORIENTED_EDGE('',*,*,#15723,.T.) ;
#20541=ORIENTED_EDGE('',*,*,#15743,.T.) ;
#20542=ORIENTED_EDGE('',*,*,#15744,.T.) ;
#20543=ORIENTED_EDGE('',*,*,#15704,.T.) ;
#20544=ORIENTED_EDGE('',*,*,#15745,.T.) ;
#20545=ORIENTED_EDGE('',*,*,#15746,.T.) ;
#20546=ORIENTED_EDGE('',*,*,#15747,.T.) ;
#20547=ORIENTED_EDGE('',*,*,#15745,.F.) ;
#20548=ORIENTED_EDGE('',*,*,#15703,.T.) ;
#20549=ORIENTED_EDGE('',*,*,#15748,.F.) ;
#20550=ORIENTED_EDGE('',*,*,#15749,.F.) ;
#20551=ORIENTED_EDGE('',*,*,#15676,.T.) ;
#20552=ORIENTED_EDGE('',*,*,#15750,.T.) ;
#20553=ORIENTED_EDGE('',*,*,#15740,.T.) ;
#20554=ORIENTED_EDGE('',*,*,#15751,.T.) ;
#20555=ORIENTED_EDGE('',*,*,#15750,.F.) ;
#20556=ORIENTED_EDGE('',*,*,#15675,.F.) ;
#20557=ORIENTED_EDGE('',*,*,#15752,.F.) ;
#20558=ORIENTED_EDGE('',*,*,#15741,.F.) ;
#20559=ORIENTED_EDGE('',*,*,#15753,.T.) ;
#20560=ORIENTED_EDGE('',*,*,#15754,.T.) ;
#20561=ORIENTED_EDGE('',*,*,#15755,.T.) ;
#20562=ORIENTED_EDGE('',*,*,#15756,.T.) ;
#20563=ORIENTED_EDGE('',*,*,#15755,.F.) ;
#20564=ORIENTED_EDGE('',*,*,#15757,.T.) ;
#20565=ORIENTED_EDGE('',*,*,#15699,.T.) ;
#20566=ORIENTED_EDGE('',*,*,#15667,.F.) ;
#20567=ORIENTED_EDGE('',*,*,#15758,.F.) ;
#20568=ORIENTED_EDGE('',*,*,#15759,.F.) ;
#20569=ORIENTED_EDGE('',*,*,#15760,.F.) ;
#20570=ORIENTED_EDGE('',*,*,#15693,.F.) ;
#20571=ORIENTED_EDGE('',*,*,#15700,.T.) ;
#20572=ORIENTED_EDGE('',*,*,#15757,.F.) ;
#20573=ORIENTED_EDGE('',*,*,#15754,.F.) ;
#20574=ORIENTED_EDGE('',*,*,#15761,.F.) ;
#20575=ORIENTED_EDGE('',*,*,#15762,.F.) ;
#20576=ORIENTED_EDGE('',*,*,#15720,.F.) ;
#20577=ORIENTED_EDGE('',*,*,#15726,.T.) ;
#20578=ORIENTED_EDGE('',*,*,#15763,.F.) ;
#20579=ORIENTED_EDGE('',*,*,#15764,.F.) ;
#20580=ORIENTED_EDGE('',*,*,#15765,.F.) ;
#20581=ORIENTED_EDGE('',*,*,#15766,.F.) ;
#20582=ORIENTED_EDGE('',*,*,#15767,.T.) ;
#20583=ORIENTED_EDGE('',*,*,#15768,.F.) ;
#20584=ORIENTED_EDGE('',*,*,#15769,.F.) ;
#20585=ORIENTED_EDGE('',*,*,#15770,.F.) ;
#20586=ORIENTED_EDGE('',*,*,#15771,.T.) ;
#20587=ORIENTED_EDGE('',*,*,#15772,.T.) ;
#20588=ORIENTED_EDGE('',*,*,#15773,.T.) ;
#20589=ORIENTED_EDGE('',*,*,#15774,.F.) ;
#20590=ORIENTED_EDGE('',*,*,#15775,.T.) ;
#20591=ORIENTED_EDGE('',*,*,#15776,.F.) ;
#20592=ORIENTED_EDGE('',*,*,#15777,.T.) ;
#20593=ORIENTED_EDGE('',*,*,#15778,.F.) ;
#20594=ORIENTED_EDGE('',*,*,#15779,.T.) ;
#20595=ORIENTED_EDGE('',*,*,#15780,.F.) ;
#20596=ORIENTED_EDGE('',*,*,#15781,.T.) ;
#20597=ORIENTED_EDGE('',*,*,#15782,.F.) ;
#20598=ORIENTED_EDGE('',*,*,#15783,.T.) ;
#20599=ORIENTED_EDGE('',*,*,#15784,.F.) ;
#20600=ORIENTED_EDGE('',*,*,#15785,.T.) ;
#20601=ORIENTED_EDGE('',*,*,#15786,.F.) ;
#20602=ORIENTED_EDGE('',*,*,#15787,.T.) ;
#20603=ORIENTED_EDGE('',*,*,#15788,.F.) ;
#20604=ORIENTED_EDGE('',*,*,#15789,.T.) ;
#20605=ORIENTED_EDGE('',*,*,#15790,.F.) ;
#20606=ORIENTED_EDGE('',*,*,#15791,.T.) ;
#20607=ORIENTED_EDGE('',*,*,#15792,.F.) ;
#20608=ORIENTED_EDGE('',*,*,#15793,.T.) ;
#20609=ORIENTED_EDGE('',*,*,#15794,.F.) ;
#20610=ORIENTED_EDGE('',*,*,#15795,.T.) ;
#20611=ORIENTED_EDGE('',*,*,#15796,.F.) ;
#20612=ORIENTED_EDGE('',*,*,#15797,.T.) ;
#20613=ORIENTED_EDGE('',*,*,#15798,.T.) ;
#20614=ORIENTED_EDGE('',*,*,#15799,.T.) ;
#20615=ORIENTED_EDGE('',*,*,#15800,.T.) ;
#20616=ORIENTED_EDGE('',*,*,#15801,.T.) ;
#20617=ORIENTED_EDGE('',*,*,#15802,.F.) ;
#20618=ORIENTED_EDGE('',*,*,#15803,.T.) ;
#20619=ORIENTED_EDGE('',*,*,#15804,.F.) ;
#20620=ORIENTED_EDGE('',*,*,#15805,.F.) ;
#20621=ORIENTED_EDGE('',*,*,#15806,.T.) ;
#20622=ORIENTED_EDGE('',*,*,#15807,.F.) ;
#20623=ORIENTED_EDGE('',*,*,#15808,.T.) ;
#20624=ORIENTED_EDGE('',*,*,#15809,.F.) ;
#20625=ORIENTED_EDGE('',*,*,#15810,.T.) ;
#20626=ORIENTED_EDGE('',*,*,#15811,.F.) ;
#20627=ORIENTED_EDGE('',*,*,#15812,.T.) ;
#20628=ORIENTED_EDGE('',*,*,#15813,.F.) ;
#20629=ORIENTED_EDGE('',*,*,#15814,.T.) ;
#20630=ORIENTED_EDGE('',*,*,#15815,.F.) ;
#20631=ORIENTED_EDGE('',*,*,#15816,.T.) ;
#20632=ORIENTED_EDGE('',*,*,#15817,.T.) ;
#20633=ORIENTED_EDGE('',*,*,#15818,.F.) ;
#20634=ORIENTED_EDGE('',*,*,#15819,.F.) ;
#20635=ORIENTED_EDGE('',*,*,#15820,.F.) ;
#20636=ORIENTED_EDGE('',*,*,#15821,.T.) ;
#20637=ORIENTED_EDGE('',*,*,#15822,.F.) ;
#20638=ORIENTED_EDGE('',*,*,#15823,.F.) ;
#20639=ORIENTED_EDGE('',*,*,#15824,.F.) ;
#20640=ORIENTED_EDGE('',*,*,#15825,.T.) ;
#20641=ORIENTED_EDGE('',*,*,#15826,.F.) ;
#20642=ORIENTED_EDGE('',*,*,#15827,.F.) ;
#20643=ORIENTED_EDGE('',*,*,#15828,.F.) ;
#20644=ORIENTED_EDGE('',*,*,#15599,.F.) ;
#20645=ORIENTED_EDGE('',*,*,#15698,.T.) ;
#20646=ORIENTED_EDGE('',*,*,#15829,.F.) ;
#20647=ORIENTED_EDGE('',*,*,#15830,.F.) ;
#20648=ORIENTED_EDGE('',*,*,#15831,.F.) ;
#20649=ORIENTED_EDGE('',*,*,#15832,.T.) ;
#20650=ORIENTED_EDGE('',*,*,#15833,.F.) ;
#20651=ORIENTED_EDGE('',*,*,#15834,.T.) ;
#20652=ORIENTED_EDGE('',*,*,#15835,.F.) ;
#20653=ORIENTED_EDGE('',*,*,#15836,.T.) ;
#20654=ORIENTED_EDGE('',*,*,#15837,.F.) ;
#20655=ORIENTED_EDGE('',*,*,#15838,.T.) ;
#20656=ORIENTED_EDGE('',*,*,#15839,.F.) ;
#20657=ORIENTED_EDGE('',*,*,#15840,.T.) ;
#20658=ORIENTED_EDGE('',*,*,#15746,.F.) ;
#20659=ORIENTED_EDGE('',*,*,#15749,.T.) ;
#20660=ORIENTED_EDGE('',*,*,#15841,.F.) ;
#20661=ORIENTED_EDGE('',*,*,#15842,.T.) ;
#20662=ORIENTED_EDGE('',*,*,#15843,.F.) ;
#20663=ORIENTED_EDGE('',*,*,#15844,.T.) ;
#20664=ORIENTED_EDGE('',*,*,#15669,.F.) ;
#20665=ORIENTED_EDGE('',*,*,#15845,.T.) ;
#20666=ORIENTED_EDGE('',*,*,#15846,.F.) ;
#20667=ORIENTED_EDGE('',*,*,#15847,.T.) ;
#20668=ORIENTED_EDGE('',*,*,#15848,.F.) ;
#20669=ORIENTED_EDGE('',*,*,#15758,.T.) ;
#20670=ORIENTED_EDGE('',*,*,#15666,.T.) ;
#20671=ORIENTED_EDGE('',*,*,#15849,.T.) ;
#20672=ORIENTED_EDGE('',*,*,#15768,.T.) ;
#20673=ORIENTED_EDGE('',*,*,#15850,.F.) ;
#20674=ORIENTED_EDGE('',*,*,#15849,.F.) ;
#20675=ORIENTED_EDGE('',*,*,#15665,.F.) ;
#20676=ORIENTED_EDGE('',*,*,#15851,.F.) ;
#20677=ORIENTED_EDGE('',*,*,#15769,.T.) ;
#20678=ORIENTED_EDGE('',*,*,#15820,.T.) ;
#20679=ORIENTED_EDGE('',*,*,#15852,.T.) ;
#20680=ORIENTED_EDGE('',*,*,#15613,.T.) ;
#20681=ORIENTED_EDGE('',*,*,#15853,.T.) ;
#20682=ORIENTED_EDGE('',*,*,#15852,.F.) ;
#20683=ORIENTED_EDGE('',*,*,#15819,.T.) ;
#20684=ORIENTED_EDGE('',*,*,#15854,.F.) ;
#20685=ORIENTED_EDGE('',*,*,#15614,.F.) ;
#20686=ORIENTED_EDGE('',*,*,#15615,.T.) ;
#20687=ORIENTED_EDGE('',*,*,#15854,.T.) ;
#20688=ORIENTED_EDGE('',*,*,#15818,.T.) ;
#20689=ORIENTED_EDGE('',*,*,#15855,.F.) ;
#20690=ORIENTED_EDGE('',*,*,#15824,.T.) ;
#20691=ORIENTED_EDGE('',*,*,#15856,.T.) ;
#20692=ORIENTED_EDGE('',*,*,#15609,.T.) ;
#20693=ORIENTED_EDGE('',*,*,#15857,.T.) ;
#20694=ORIENTED_EDGE('',*,*,#15856,.F.) ;
#20695=ORIENTED_EDGE('',*,*,#15823,.T.) ;
#20696=ORIENTED_EDGE('',*,*,#15858,.F.) ;
#20697=ORIENTED_EDGE('',*,*,#15610,.F.) ;
#20698=ORIENTED_EDGE('',*,*,#15611,.T.) ;
#20699=ORIENTED_EDGE('',*,*,#15858,.T.) ;
#20700=ORIENTED_EDGE('',*,*,#15822,.T.) ;
#20701=ORIENTED_EDGE('',*,*,#15859,.F.) ;
#20702=ORIENTED_EDGE('',*,*,#15828,.T.) ;
#20703=ORIENTED_EDGE('',*,*,#15860,.T.) ;
#20704=ORIENTED_EDGE('',*,*,#15606,.T.) ;
#20705=ORIENTED_EDGE('',*,*,#15861,.T.) ;
#20706=ORIENTED_EDGE('',*,*,#15860,.F.) ;
#20707=ORIENTED_EDGE('',*,*,#15827,.T.) ;
#20708=ORIENTED_EDGE('',*,*,#15862,.F.) ;
#20709=ORIENTED_EDGE('',*,*,#15607,.F.) ;
#20710=ORIENTED_EDGE('',*,*,#15608,.T.) ;
#20711=ORIENTED_EDGE('',*,*,#15862,.T.) ;
#20712=ORIENTED_EDGE('',*,*,#15826,.T.) ;
#20713=ORIENTED_EDGE('',*,*,#15863,.F.) ;
#20714=ORIENTED_EDGE('',*,*,#15770,.T.) ;
#20715=ORIENTED_EDGE('',*,*,#15851,.T.) ;
#20716=ORIENTED_EDGE('',*,*,#15664,.T.) ;
#20717=ORIENTED_EDGE('',*,*,#15864,.T.) ;
#20718=ORIENTED_EDGE('',*,*,#15848,.T.) ;
#20719=ORIENTED_EDGE('',*,*,#15865,.T.) ;
#20720=ORIENTED_EDGE('',*,*,#15866,.T.) ;
#20721=ORIENTED_EDGE('',*,*,#15759,.T.) ;
#20722=ORIENTED_EDGE('',*,*,#15865,.F.) ;
#20723=ORIENTED_EDGE('',*,*,#15847,.F.) ;
#20724=ORIENTED_EDGE('',*,*,#15867,.F.) ;
#20725=ORIENTED_EDGE('',*,*,#15868,.F.) ;
#20726=ORIENTED_EDGE('',*,*,#15846,.T.) ;
#20727=ORIENTED_EDGE('',*,*,#15869,.T.) ;
#20728=ORIENTED_EDGE('',*,*,#15870,.T.) ;
#20729=ORIENTED_EDGE('',*,*,#15867,.T.) ;
#20730=ORIENTED_EDGE('',*,*,#15753,.F.) ;
#20731=ORIENTED_EDGE('',*,*,#15871,.T.) ;
#20732=ORIENTED_EDGE('',*,*,#15869,.F.) ;
#20733=ORIENTED_EDGE('',*,*,#15845,.F.) ;
#20734=ORIENTED_EDGE('',*,*,#15668,.F.) ;
#20735=ORIENTED_EDGE('',*,*,#15872,.F.) ;
#20736=ORIENTED_EDGE('',*,*,#15761,.T.) ;
#20737=ORIENTED_EDGE('',*,*,#15674,.T.) ;
#20738=ORIENTED_EDGE('',*,*,#15724,.T.) ;
#20739=ORIENTED_EDGE('',*,*,#15742,.T.) ;
#20740=ORIENTED_EDGE('',*,*,#15752,.T.) ;
#20741=ORIENTED_EDGE('',*,*,#15873,.T.) ;
#20742=ORIENTED_EDGE('',*,*,#15874,.T.) ;
#20743=ORIENTED_EDGE('',*,*,#15875,.T.) ;
#20744=ORIENTED_EDGE('',*,*,#15876,.T.) ;
#20745=ORIENTED_EDGE('',*,*,#15874,.F.) ;
#20746=ORIENTED_EDGE('',*,*,#15877,.T.) ;
#20747=ORIENTED_EDGE('',*,*,#15878,.F.) ;
#20748=ORIENTED_EDGE('',*,*,#15879,.T.) ;
#20749=ORIENTED_EDGE('',*,*,#15873,.F.) ;
#20750=ORIENTED_EDGE('',*,*,#15880,.T.) ;
#20751=ORIENTED_EDGE('',*,*,#15881,.F.) ;
#20752=ORIENTED_EDGE('',*,*,#15882,.T.) ;
#20753=ORIENTED_EDGE('',*,*,#15883,.F.) ;
#20754=ORIENTED_EDGE('',*,*,#15877,.F.) ;
#20755=ORIENTED_EDGE('',*,*,#15884,.T.) ;
#20756=ORIENTED_EDGE('',*,*,#15878,.T.) ;
#20757=ORIENTED_EDGE('',*,*,#15883,.T.) ;
#20758=ORIENTED_EDGE('',*,*,#15885,.T.) ;
#20759=ORIENTED_EDGE('',*,*,#15886,.T.) ;
#20760=ORIENTED_EDGE('',*,*,#15887,.T.) ;
#20761=ORIENTED_EDGE('',*,*,#15885,.F.) ;
#20762=ORIENTED_EDGE('',*,*,#15882,.F.) ;
#20763=ORIENTED_EDGE('',*,*,#15888,.F.) ;
#20764=ORIENTED_EDGE('',*,*,#15889,.F.) ;
#20765=ORIENTED_EDGE('',*,*,#15765,.T.) ;
#20766=ORIENTED_EDGE('',*,*,#15841,.T.) ;
#20767=ORIENTED_EDGE('',*,*,#15748,.T.) ;
#20768=ORIENTED_EDGE('',*,*,#15702,.T.) ;
#20769=ORIENTED_EDGE('',*,*,#15890,.T.) ;
#20770=ORIENTED_EDGE('',*,*,#15694,.F.) ;
#20771=ORIENTED_EDGE('',*,*,#15766,.T.) ;
#20772=ORIENTED_EDGE('',*,*,#15889,.T.) ;
#20773=ORIENTED_EDGE('',*,*,#15596,.F.) ;
#20774=ORIENTED_EDGE('',*,*,#15842,.F.) ;
#20775=ORIENTED_EDGE('',*,*,#15890,.F.) ;
#20776=ORIENTED_EDGE('',*,*,#15701,.F.) ;
#20777=ORIENTED_EDGE('',*,*,#15738,.T.) ;
#20778=ORIENTED_EDGE('',*,*,#15891,.T.) ;
#20779=ORIENTED_EDGE('',*,*,#15678,.T.) ;
#20780=ORIENTED_EDGE('',*,*,#15892,.T.) ;
#20781=ORIENTED_EDGE('',*,*,#15891,.F.) ;
#20782=ORIENTED_EDGE('',*,*,#15737,.T.) ;
#20783=ORIENTED_EDGE('',*,*,#15893,.F.) ;
#20784=ORIENTED_EDGE('',*,*,#15679,.T.) ;
#20785=ORIENTED_EDGE('',*,*,#15682,.T.) ;
#20786=ORIENTED_EDGE('',*,*,#15894,.T.) ;
#20787=ORIENTED_EDGE('',*,*,#15734,.T.) ;
#20788=ORIENTED_EDGE('',*,*,#15895,.T.) ;
#20789=ORIENTED_EDGE('',*,*,#15894,.F.) ;
#20790=ORIENTED_EDGE('',*,*,#15681,.F.) ;
#20791=ORIENTED_EDGE('',*,*,#15896,.F.) ;
#20792=ORIENTED_EDGE('',*,*,#15735,.F.) ;
#20793=ORIENTED_EDGE('',*,*,#15680,.T.) ;
#20794=ORIENTED_EDGE('',*,*,#15893,.T.) ;
#20795=ORIENTED_EDGE('',*,*,#15736,.T.) ;
#20796=ORIENTED_EDGE('',*,*,#15896,.T.) ;
#20797=ORIENTED_EDGE('',*,*,#15730,.T.) ;
#20798=ORIENTED_EDGE('',*,*,#15897,.T.) ;
#20799=ORIENTED_EDGE('',*,*,#15686,.T.) ;
#20800=ORIENTED_EDGE('',*,*,#15898,.T.) ;
#20801=ORIENTED_EDGE('',*,*,#15897,.F.) ;
#20802=ORIENTED_EDGE('',*,*,#15729,.T.) ;
#20803=ORIENTED_EDGE('',*,*,#15899,.F.) ;
#20804=ORIENTED_EDGE('',*,*,#15687,.T.) ;
#20805=ORIENTED_EDGE('',*,*,#15684,.T.) ;
#20806=ORIENTED_EDGE('',*,*,#15900,.T.) ;
#20807=ORIENTED_EDGE('',*,*,#15732,.T.) ;
#20808=ORIENTED_EDGE('',*,*,#15901,.T.) ;
#20809=ORIENTED_EDGE('',*,*,#15895,.F.) ;
#20810=ORIENTED_EDGE('',*,*,#15733,.F.) ;
#20811=ORIENTED_EDGE('',*,*,#15900,.F.) ;
#20812=ORIENTED_EDGE('',*,*,#15683,.F.) ;
#20813=ORIENTED_EDGE('',*,*,#15688,.T.) ;
#20814=ORIENTED_EDGE('',*,*,#15899,.T.) ;
#20815=ORIENTED_EDGE('',*,*,#15728,.T.) ;
#20816=ORIENTED_EDGE('',*,*,#15902,.T.) ;
#20817=ORIENTED_EDGE('',*,*,#15833,.T.) ;
#20818=ORIENTED_EDGE('',*,*,#15903,.T.) ;
#20819=ORIENTED_EDGE('',*,*,#15712,.T.) ;
#20820=ORIENTED_EDGE('',*,*,#15904,.T.) ;
#20821=ORIENTED_EDGE('',*,*,#15903,.F.) ;
#20822=ORIENTED_EDGE('',*,*,#15832,.F.) ;
#20823=ORIENTED_EDGE('',*,*,#15905,.F.) ;
#20824=ORIENTED_EDGE('',*,*,#15713,.F.) ;
#20825=ORIENTED_EDGE('',*,*,#15831,.T.) ;
#20826=ORIENTED_EDGE('',*,*,#15906,.T.) ;
#20827=ORIENTED_EDGE('',*,*,#15714,.T.) ;
#20828=ORIENTED_EDGE('',*,*,#15905,.T.) ;
#20829=ORIENTED_EDGE('',*,*,#15906,.F.) ;
#20830=ORIENTED_EDGE('',*,*,#15830,.T.) ;
#20831=ORIENTED_EDGE('',*,*,#15907,.F.) ;
#20832=ORIENTED_EDGE('',*,*,#15715,.T.) ;
#20833=ORIENTED_EDGE('',*,*,#15716,.T.) ;
#20834=ORIENTED_EDGE('',*,*,#15907,.T.) ;
#20835=ORIENTED_EDGE('',*,*,#15829,.T.) ;
#20836=ORIENTED_EDGE('',*,*,#15697,.T.) ;
#20837=ORIENTED_EDGE('',*,*,#15710,.T.) ;
#20838=ORIENTED_EDGE('',*,*,#15908,.T.) ;
#20839=ORIENTED_EDGE('',*,*,#15835,.T.) ;
#20840=ORIENTED_EDGE('',*,*,#15909,.T.) ;
#20841=ORIENTED_EDGE('',*,*,#15908,.F.) ;
#20842=ORIENTED_EDGE('',*,*,#15709,.T.) ;
#20843=ORIENTED_EDGE('',*,*,#15910,.F.) ;
#20844=ORIENTED_EDGE('',*,*,#15836,.F.) ;
#20845=ORIENTED_EDGE('',*,*,#15837,.T.) ;
#20846=ORIENTED_EDGE('',*,*,#15910,.T.) ;
#20847=ORIENTED_EDGE('',*,*,#15708,.T.) ;
#20848=ORIENTED_EDGE('',*,*,#15911,.T.) ;
#20849=ORIENTED_EDGE('',*,*,#15747,.F.) ;
#20850=ORIENTED_EDGE('',*,*,#15840,.F.) ;
#20851=ORIENTED_EDGE('',*,*,#15912,.F.) ;
#20852=ORIENTED_EDGE('',*,*,#15705,.T.) ;
#20853=ORIENTED_EDGE('',*,*,#15839,.T.) ;
#20854=ORIENTED_EDGE('',*,*,#15913,.T.) ;
#20855=ORIENTED_EDGE('',*,*,#15706,.T.) ;
#20856=ORIENTED_EDGE('',*,*,#15912,.T.) ;
#20857=ORIENTED_EDGE('',*,*,#15911,.F.) ;
#20858=ORIENTED_EDGE('',*,*,#15707,.T.) ;
#20859=ORIENTED_EDGE('',*,*,#15913,.F.) ;
#20860=ORIENTED_EDGE('',*,*,#15838,.F.) ;
#20861=ORIENTED_EDGE('',*,*,#15888,.T.) ;
#20862=ORIENTED_EDGE('',*,*,#15881,.T.) ;
#20863=ORIENTED_EDGE('',*,*,#15914,.T.) ;
#20864=ORIENTED_EDGE('',*,*,#15600,.T.) ;
#20865=ORIENTED_EDGE('',*,*,#15914,.F.) ;
#20866=ORIENTED_EDGE('',*,*,#15880,.F.) ;
#20867=ORIENTED_EDGE('',*,*,#15876,.F.) ;
#20868=ORIENTED_EDGE('',*,*,#15915,.F.) ;
#20869=ORIENTED_EDGE('',*,*,#15916,.T.) ;
#20870=ORIENTED_EDGE('',*,*,#15763,.T.) ;
#20871=ORIENTED_EDGE('',*,*,#15725,.T.) ;
#20872=ORIENTED_EDGE('',*,*,#15721,.F.) ;
#20873=ORIENTED_EDGE('',*,*,#15762,.T.) ;
#20874=ORIENTED_EDGE('',*,*,#15872,.T.) ;
#20875=ORIENTED_EDGE('',*,*,#15602,.F.) ;
#20876=ORIENTED_EDGE('',*,*,#15672,.F.) ;
#20877=ORIENTED_EDGE('',*,*,#15689,.F.) ;
#20878=ORIENTED_EDGE('',*,*,#15902,.F.) ;
#20879=ORIENTED_EDGE('',*,*,#15727,.T.) ;
#20880=ORIENTED_EDGE('',*,*,#15751,.F.) ;
#20881=ORIENTED_EDGE('',*,*,#15739,.F.) ;
#20882=ORIENTED_EDGE('',*,*,#15892,.F.) ;
#20883=ORIENTED_EDGE('',*,*,#15677,.F.) ;
#20884=ORIENTED_EDGE('',*,*,#15691,.F.) ;
#20885=ORIENTED_EDGE('',*,*,#15917,.T.) ;
#20886=ORIENTED_EDGE('',*,*,#15744,.F.) ;
#20887=ORIENTED_EDGE('',*,*,#15917,.F.) ;
#20888=ORIENTED_EDGE('',*,*,#15690,.F.) ;
#20889=ORIENTED_EDGE('',*,*,#15918,.T.) ;
#20890=ORIENTED_EDGE('',*,*,#15743,.F.) ;
#20891=ORIENTED_EDGE('',*,*,#15918,.F.) ;
#20892=ORIENTED_EDGE('',*,*,#15898,.F.) ;
#20893=ORIENTED_EDGE('',*,*,#15685,.F.) ;
#20894=ORIENTED_EDGE('',*,*,#15901,.F.) ;
#20895=ORIENTED_EDGE('',*,*,#15731,.F.) ;
#20896=ORIENTED_EDGE('',*,*,#15718,.F.) ;
#20897=ORIENTED_EDGE('',*,*,#15919,.T.) ;
#20898=ORIENTED_EDGE('',*,*,#15844,.F.) ;
#20899=ORIENTED_EDGE('',*,*,#15919,.F.) ;
#20900=ORIENTED_EDGE('',*,*,#15618,.T.) ;
#20901=ORIENTED_EDGE('',*,*,#15920,.F.) ;
#20902=ORIENTED_EDGE('',*,*,#15804,.T.) ;
#20903=ORIENTED_EDGE('',*,*,#15921,.T.) ;
#20904=ORIENTED_EDGE('',*,*,#15620,.T.) ;
#20905=ORIENTED_EDGE('',*,*,#15922,.F.) ;
#20906=ORIENTED_EDGE('',*,*,#15802,.T.) ;
#20907=ORIENTED_EDGE('',*,*,#15923,.F.) ;
#20908=ORIENTED_EDGE('',*,*,#15801,.F.) ;
#20909=ORIENTED_EDGE('',*,*,#15920,.T.) ;
#20910=ORIENTED_EDGE('',*,*,#15617,.F.) ;
#20911=ORIENTED_EDGE('',*,*,#15923,.T.) ;
#20912=ORIENTED_EDGE('',*,*,#15803,.F.) ;
#20913=ORIENTED_EDGE('',*,*,#15922,.T.) ;
#20914=ORIENTED_EDGE('',*,*,#15619,.F.) ;
#20915=ORIENTED_EDGE('',*,*,#15921,.F.) ;
#20916=ORIENTED_EDGE('',*,*,#15821,.F.) ;
#20917=ORIENTED_EDGE('',*,*,#15857,.F.) ;
#20918=ORIENTED_EDGE('',*,*,#15612,.F.) ;
#20919=ORIENTED_EDGE('',*,*,#15859,.T.) ;
#20920=ORIENTED_EDGE('',*,*,#15646,.F.) ;
#20921=ORIENTED_EDGE('',*,*,#15924,.T.) ;
#20922=ORIENTED_EDGE('',*,*,#15771,.F.) ;
#20923=ORIENTED_EDGE('',*,*,#15924,.F.) ;
#20924=ORIENTED_EDGE('',*,*,#15645,.F.) ;
#20925=ORIENTED_EDGE('',*,*,#15925,.T.) ;
#20926=ORIENTED_EDGE('',*,*,#15772,.F.) ;
#20927=ORIENTED_EDGE('',*,*,#15925,.F.) ;
#20928=ORIENTED_EDGE('',*,*,#15904,.F.) ;
#20929=ORIENTED_EDGE('',*,*,#15711,.T.) ;
#20930=ORIENTED_EDGE('',*,*,#15909,.F.) ;
#20931=ORIENTED_EDGE('',*,*,#15834,.F.) ;
#20932=ORIENTED_EDGE('',*,*,#15756,.F.) ;
#20933=ORIENTED_EDGE('',*,*,#15760,.T.) ;
#20934=ORIENTED_EDGE('',*,*,#15866,.F.) ;
#20935=ORIENTED_EDGE('',*,*,#15868,.T.) ;
#20936=ORIENTED_EDGE('',*,*,#15870,.F.) ;
#20937=ORIENTED_EDGE('',*,*,#15871,.F.) ;
#20938=ORIENTED_EDGE('',*,*,#15647,.F.) ;
#20939=ORIENTED_EDGE('',*,*,#15926,.T.) ;
#20940=ORIENTED_EDGE('',*,*,#15800,.F.) ;
#20941=ORIENTED_EDGE('',*,*,#15926,.F.) ;
#20942=ORIENTED_EDGE('',*,*,#15648,.F.) ;
#20943=ORIENTED_EDGE('',*,*,#15927,.T.) ;
#20944=ORIENTED_EDGE('',*,*,#15799,.F.) ;
#20945=ORIENTED_EDGE('',*,*,#15927,.F.) ;
#20946=ORIENTED_EDGE('',*,*,#15649,.F.) ;
#20947=ORIENTED_EDGE('',*,*,#15928,.T.) ;
#20948=ORIENTED_EDGE('',*,*,#15798,.F.) ;
#20949=ORIENTED_EDGE('',*,*,#15928,.F.) ;
#20950=ORIENTED_EDGE('',*,*,#15650,.F.) ;
#20951=ORIENTED_EDGE('',*,*,#15929,.T.) ;
#20952=ORIENTED_EDGE('',*,*,#15797,.F.) ;
#20953=ORIENTED_EDGE('',*,*,#15929,.F.) ;
#20954=ORIENTED_EDGE('',*,*,#15795,.F.) ;
#20955=ORIENTED_EDGE('',*,*,#15930,.T.) ;
#20956=ORIENTED_EDGE('',*,*,#15642,.F.) ;
#20957=ORIENTED_EDGE('',*,*,#15931,.T.) ;
#20958=ORIENTED_EDGE('',*,*,#15794,.T.) ;
#20959=ORIENTED_EDGE('',*,*,#15932,.F.) ;
#20960=ORIENTED_EDGE('',*,*,#15643,.T.) ;
#20961=ORIENTED_EDGE('',*,*,#15930,.F.) ;
#20962=ORIENTED_EDGE('',*,*,#15793,.F.) ;
#20963=ORIENTED_EDGE('',*,*,#15933,.T.) ;
#20964=ORIENTED_EDGE('',*,*,#15644,.F.) ;
#20965=ORIENTED_EDGE('',*,*,#15932,.T.) ;
#20966=ORIENTED_EDGE('',*,*,#15796,.T.) ;
#20967=ORIENTED_EDGE('',*,*,#15931,.F.) ;
#20968=ORIENTED_EDGE('',*,*,#15641,.T.) ;
#20969=ORIENTED_EDGE('',*,*,#15933,.F.) ;
#20970=ORIENTED_EDGE('',*,*,#15791,.F.) ;
#20971=ORIENTED_EDGE('',*,*,#15934,.T.) ;
#20972=ORIENTED_EDGE('',*,*,#15638,.F.) ;
#20973=ORIENTED_EDGE('',*,*,#15935,.T.) ;
#20974=ORIENTED_EDGE('',*,*,#15790,.T.) ;
#20975=ORIENTED_EDGE('',*,*,#15936,.F.) ;
#20976=ORIENTED_EDGE('',*,*,#15639,.T.) ;
#20977=ORIENTED_EDGE('',*,*,#15934,.F.) ;
#20978=ORIENTED_EDGE('',*,*,#15789,.F.) ;
#20979=ORIENTED_EDGE('',*,*,#15937,.T.) ;
#20980=ORIENTED_EDGE('',*,*,#15640,.F.) ;
#20981=ORIENTED_EDGE('',*,*,#15936,.T.) ;
#20982=ORIENTED_EDGE('',*,*,#15792,.T.) ;
#20983=ORIENTED_EDGE('',*,*,#15935,.F.) ;
#20984=ORIENTED_EDGE('',*,*,#15637,.T.) ;
#20985=ORIENTED_EDGE('',*,*,#15937,.F.) ;
#20986=ORIENTED_EDGE('',*,*,#15787,.F.) ;
#20987=ORIENTED_EDGE('',*,*,#15938,.T.) ;
#20988=ORIENTED_EDGE('',*,*,#15634,.F.) ;
#20989=ORIENTED_EDGE('',*,*,#15939,.T.) ;
#20990=ORIENTED_EDGE('',*,*,#15786,.T.) ;
#20991=ORIENTED_EDGE('',*,*,#15940,.F.) ;
#20992=ORIENTED_EDGE('',*,*,#15635,.T.) ;
#20993=ORIENTED_EDGE('',*,*,#15938,.F.) ;
#20994=ORIENTED_EDGE('',*,*,#15785,.F.) ;
#20995=ORIENTED_EDGE('',*,*,#15941,.T.) ;
#20996=ORIENTED_EDGE('',*,*,#15636,.F.) ;
#20997=ORIENTED_EDGE('',*,*,#15940,.T.) ;
#20998=ORIENTED_EDGE('',*,*,#15788,.T.) ;
#20999=ORIENTED_EDGE('',*,*,#15939,.F.) ;
#21000=ORIENTED_EDGE('',*,*,#15633,.T.) ;
#21001=ORIENTED_EDGE('',*,*,#15941,.F.) ;
#21002=ORIENTED_EDGE('',*,*,#15783,.F.) ;
#21003=ORIENTED_EDGE('',*,*,#15942,.T.) ;
#21004=ORIENTED_EDGE('',*,*,#15630,.F.) ;
#21005=ORIENTED_EDGE('',*,*,#15943,.T.) ;
#21006=ORIENTED_EDGE('',*,*,#15782,.T.) ;
#21007=ORIENTED_EDGE('',*,*,#15944,.F.) ;
#21008=ORIENTED_EDGE('',*,*,#15631,.T.) ;
#21009=ORIENTED_EDGE('',*,*,#15942,.F.) ;
#21010=ORIENTED_EDGE('',*,*,#15781,.F.) ;
#21011=ORIENTED_EDGE('',*,*,#15945,.T.) ;
#21012=ORIENTED_EDGE('',*,*,#15632,.F.) ;
#21013=ORIENTED_EDGE('',*,*,#15944,.T.) ;
#21014=ORIENTED_EDGE('',*,*,#15784,.T.) ;
#21015=ORIENTED_EDGE('',*,*,#15943,.F.) ;
#21016=ORIENTED_EDGE('',*,*,#15629,.T.) ;
#21017=ORIENTED_EDGE('',*,*,#15945,.F.) ;
#21018=ORIENTED_EDGE('',*,*,#15779,.F.) ;
#21019=ORIENTED_EDGE('',*,*,#15946,.T.) ;
#21020=ORIENTED_EDGE('',*,*,#15626,.F.) ;
#21021=ORIENTED_EDGE('',*,*,#15947,.T.) ;
#21022=ORIENTED_EDGE('',*,*,#15778,.T.) ;
#21023=ORIENTED_EDGE('',*,*,#15948,.F.) ;
#21024=ORIENTED_EDGE('',*,*,#15627,.T.) ;
#21025=ORIENTED_EDGE('',*,*,#15946,.F.) ;
#21026=ORIENTED_EDGE('',*,*,#15777,.F.) ;
#21027=ORIENTED_EDGE('',*,*,#15949,.T.) ;
#21028=ORIENTED_EDGE('',*,*,#15628,.F.) ;
#21029=ORIENTED_EDGE('',*,*,#15948,.T.) ;
#21030=ORIENTED_EDGE('',*,*,#15780,.T.) ;
#21031=ORIENTED_EDGE('',*,*,#15947,.F.) ;
#21032=ORIENTED_EDGE('',*,*,#15625,.T.) ;
#21033=ORIENTED_EDGE('',*,*,#15949,.F.) ;
#21034=ORIENTED_EDGE('',*,*,#15775,.F.) ;
#21035=ORIENTED_EDGE('',*,*,#15950,.T.) ;
#21036=ORIENTED_EDGE('',*,*,#15622,.F.) ;
#21037=ORIENTED_EDGE('',*,*,#15951,.T.) ;
#21038=ORIENTED_EDGE('',*,*,#15774,.T.) ;
#21039=ORIENTED_EDGE('',*,*,#15952,.F.) ;
#21040=ORIENTED_EDGE('',*,*,#15623,.T.) ;
#21041=ORIENTED_EDGE('',*,*,#15950,.F.) ;
#21042=ORIENTED_EDGE('',*,*,#15773,.F.) ;
#21043=ORIENTED_EDGE('',*,*,#15953,.T.) ;
#21044=ORIENTED_EDGE('',*,*,#15624,.F.) ;
#21045=ORIENTED_EDGE('',*,*,#15952,.T.) ;
#21046=ORIENTED_EDGE('',*,*,#15776,.T.) ;
#21047=ORIENTED_EDGE('',*,*,#15951,.F.) ;
#21048=ORIENTED_EDGE('',*,*,#15621,.T.) ;
#21049=ORIENTED_EDGE('',*,*,#15953,.F.) ;
#21050=ORIENTED_EDGE('',*,*,#15764,.T.) ;
#21051=ORIENTED_EDGE('',*,*,#15916,.F.) ;
#21052=ORIENTED_EDGE('',*,*,#15954,.T.) ;
#21053=ORIENTED_EDGE('',*,*,#15886,.F.) ;
#21054=ORIENTED_EDGE('',*,*,#15875,.F.) ;
#21055=ORIENTED_EDGE('',*,*,#15879,.F.) ;
#21056=ORIENTED_EDGE('',*,*,#15884,.F.) ;
#21057=ORIENTED_EDGE('',*,*,#15887,.F.) ;
#21058=ORIENTED_EDGE('',*,*,#15954,.F.) ;
#21059=ORIENTED_EDGE('',*,*,#15915,.T.) ;
#21060=ORIENTED_EDGE('',*,*,#15717,.T.) ;
#21061=ORIENTED_EDGE('',*,*,#15955,.T.) ;
#21062=ORIENTED_EDGE('',*,*,#15843,.T.) ;
#21063=ORIENTED_EDGE('',*,*,#15955,.F.) ;
#21064=ORIENTED_EDGE('',*,*,#15825,.F.) ;
#21065=ORIENTED_EDGE('',*,*,#15861,.F.) ;
#21066=ORIENTED_EDGE('',*,*,#15605,.F.) ;
#21067=ORIENTED_EDGE('',*,*,#15863,.T.) ;
#21068=ORIENTED_EDGE('',*,*,#15767,.F.) ;
#21069=ORIENTED_EDGE('',*,*,#15864,.F.) ;
#21070=ORIENTED_EDGE('',*,*,#15663,.F.) ;
#21071=ORIENTED_EDGE('',*,*,#15850,.T.) ;
#21072=ORIENTED_EDGE('',*,*,#15817,.F.) ;
#21073=ORIENTED_EDGE('',*,*,#15853,.F.) ;
#21074=ORIENTED_EDGE('',*,*,#15616,.F.) ;
#21075=ORIENTED_EDGE('',*,*,#15855,.T.) ;
#21076=ORIENTED_EDGE('',*,*,#15651,.T.) ;
#21077=ORIENTED_EDGE('',*,*,#15956,.F.) ;
#21078=ORIENTED_EDGE('',*,*,#15805,.T.) ;
#21079=ORIENTED_EDGE('',*,*,#15957,.T.) ;
#21080=ORIENTED_EDGE('',*,*,#15653,.T.) ;
#21081=ORIENTED_EDGE('',*,*,#15958,.F.) ;
#21082=ORIENTED_EDGE('',*,*,#15807,.T.) ;
#21083=ORIENTED_EDGE('',*,*,#15959,.F.) ;
#21084=ORIENTED_EDGE('',*,*,#15806,.F.) ;
#21085=ORIENTED_EDGE('',*,*,#15956,.T.) ;
#21086=ORIENTED_EDGE('',*,*,#15654,.F.) ;
#21087=ORIENTED_EDGE('',*,*,#15959,.T.) ;
#21088=ORIENTED_EDGE('',*,*,#15808,.F.) ;
#21089=ORIENTED_EDGE('',*,*,#15958,.T.) ;
#21090=ORIENTED_EDGE('',*,*,#15652,.F.) ;
#21091=ORIENTED_EDGE('',*,*,#15957,.F.) ;
#21092=ORIENTED_EDGE('',*,*,#15655,.T.) ;
#21093=ORIENTED_EDGE('',*,*,#15960,.F.) ;
#21094=ORIENTED_EDGE('',*,*,#15809,.T.) ;
#21095=ORIENTED_EDGE('',*,*,#15961,.T.) ;
#21096=ORIENTED_EDGE('',*,*,#15657,.T.) ;
#21097=ORIENTED_EDGE('',*,*,#15962,.F.) ;
#21098=ORIENTED_EDGE('',*,*,#15811,.T.) ;
#21099=ORIENTED_EDGE('',*,*,#15963,.F.) ;
#21100=ORIENTED_EDGE('',*,*,#15810,.F.) ;
#21101=ORIENTED_EDGE('',*,*,#15960,.T.) ;
#21102=ORIENTED_EDGE('',*,*,#15658,.F.) ;
#21103=ORIENTED_EDGE('',*,*,#15963,.T.) ;
#21104=ORIENTED_EDGE('',*,*,#15812,.F.) ;
#21105=ORIENTED_EDGE('',*,*,#15962,.T.) ;
#21106=ORIENTED_EDGE('',*,*,#15656,.F.) ;
#21107=ORIENTED_EDGE('',*,*,#15961,.F.) ;
#21108=ORIENTED_EDGE('',*,*,#15659,.T.) ;
#21109=ORIENTED_EDGE('',*,*,#15964,.F.) ;
#21110=ORIENTED_EDGE('',*,*,#15813,.T.) ;
#21111=ORIENTED_EDGE('',*,*,#15965,.T.) ;
#21112=ORIENTED_EDGE('',*,*,#15661,.T.) ;
#21113=ORIENTED_EDGE('',*,*,#15966,.F.) ;
#21114=ORIENTED_EDGE('',*,*,#15815,.T.) ;
#21115=ORIENTED_EDGE('',*,*,#15967,.F.) ;
#21116=ORIENTED_EDGE('',*,*,#15814,.F.) ;
#21117=ORIENTED_EDGE('',*,*,#15964,.T.) ;
#21118=ORIENTED_EDGE('',*,*,#15662,.F.) ;
#21119=ORIENTED_EDGE('',*,*,#15967,.T.) ;
#21120=ORIENTED_EDGE('',*,*,#15816,.F.) ;
#21121=ORIENTED_EDGE('',*,*,#15966,.T.) ;
#21122=ORIENTED_EDGE('',*,*,#15660,.F.) ;
#21123=ORIENTED_EDGE('',*,*,#15965,.F.) ;
#29948=CYLINDRICAL_SURFACE('',#32774,0.25) ;
#29949=CYLINDRICAL_SURFACE('',#32826,0.25) ;
#29950=CYLINDRICAL_SURFACE('',#32829,0.25) ;
#29951=CYLINDRICAL_SURFACE('',#32843,0.75) ;
#29952=CYLINDRICAL_SURFACE('',#32858,0.75) ;
#29953=CYLINDRICAL_SURFACE('',#32873,1.) ;
#29954=CYLINDRICAL_SURFACE('',#32876,1.) ;
#29955=CYLINDRICAL_SURFACE('',#32878,0.75) ;
#29956=CYLINDRICAL_SURFACE('',#32944,2.4999999999) ;
#29957=CYLINDRICAL_SURFACE('',#32945,28.5) ;
#29958=CYLINDRICAL_SURFACE('',#32946,2.4999999999) ;
#29959=CYLINDRICAL_SURFACE('',#32947,28.5) ;
#29960=CYLINDRICAL_SURFACE('',#32948,2.4999999999) ;
#29961=CYLINDRICAL_SURFACE('',#32949,28.5) ;
#29962=CYLINDRICAL_SURFACE('',#32950,2.4999999999) ;
#29963=CYLINDRICAL_SURFACE('',#32951,28.5) ;
#29964=CYLINDRICAL_SURFACE('',#32952,2.4999999999) ;
#29965=CYLINDRICAL_SURFACE('',#32953,2.4999999999) ;
#29966=CYLINDRICAL_SURFACE('',#32954,0.5) ;
#29967=CYLINDRICAL_SURFACE('',#32957,0.5) ;
#29968=CYLINDRICAL_SURFACE('',#32960,0.5) ;
#29969=CYLINDRICAL_SURFACE('',#32961,0.5) ;
#29970=CYLINDRICAL_SURFACE('',#32967,0.5) ;
#29971=CYLINDRICAL_SURFACE('',#32972,0.5) ;
#29972=CYLINDRICAL_SURFACE('',#32974,1.) ;
#29973=CYLINDRICAL_SURFACE('',#32976,1.) ;
#29974=CYLINDRICAL_SURFACE('',#32978,1.) ;
#29975=CYLINDRICAL_SURFACE('',#32979,1.) ;
#29976=CYLINDRICAL_SURFACE('',#32981,1.) ;
#29977=CYLINDRICAL_SURFACE('',#32983,1.) ;
#29978=CYLINDRICAL_SURFACE('',#32984,1.) ;
#29979=CYLINDRICAL_SURFACE('',#32986,1.) ;
#29980=CYLINDRICAL_SURFACE('',#32988,1.) ;
#29981=CYLINDRICAL_SURFACE('',#32989,1.) ;
#29982=CYLINDRICAL_SURFACE('',#32991,1.) ;
#29983=CYLINDRICAL_SURFACE('',#32993,1.) ;
#29984=CYLINDRICAL_SURFACE('',#32995,0.25) ;
#29985=CYLINDRICAL_SURFACE('',#33001,1.25) ;
#29986=CYLINDRICAL_SURFACE('',#33002,1.25) ;
#29987=CYLINDRICAL_SURFACE('',#33004,1.25) ;
#29988=CYLINDRICAL_SURFACE('',#33005,3.) ;
#29989=CYLINDRICAL_SURFACE('',#33006,3.) ;
#29990=CYLINDRICAL_SURFACE('',#33007,15.5) ;
#29991=CYLINDRICAL_SURFACE('',#33008,21.5) ;
#29992=CYLINDRICAL_SURFACE('',#33009,23.5) ;
#29993=CYLINDRICAL_SURFACE('',#33014,2.) ;
#29994=CYLINDRICAL_SURFACE('',#33015,2.) ;
#29995=CYLINDRICAL_SURFACE('',#33016,2.) ;
#29996=CYLINDRICAL_SURFACE('',#33017,2.) ;
#29997=CYLINDRICAL_SURFACE('',#33018,1.5) ;
#29998=CYLINDRICAL_SURFACE('',#33020,1.5) ;
#29999=CYLINDRICAL_SURFACE('',#33022,1.5) ;
#30000=CYLINDRICAL_SURFACE('',#33024,1.5) ;
#30001=CYLINDRICAL_SURFACE('',#33026,1.5) ;
#30002=CYLINDRICAL_SURFACE('',#33028,1.5) ;
#30003=CYLINDRICAL_SURFACE('',#33030,1.5) ;
#30004=CYLINDRICAL_SURFACE('',#33032,1.5) ;
#30005=CYLINDRICAL_SURFACE('',#33034,1.5) ;
#30006=CYLINDRICAL_SURFACE('',#33036,1.5) ;
#30007=CYLINDRICAL_SURFACE('',#33038,1.5) ;
#30008=CYLINDRICAL_SURFACE('',#33040,1.5) ;
#30009=CYLINDRICAL_SURFACE('',#33042,0.75) ;
#30010=CYLINDRICAL_SURFACE('',#33044,1.25) ;
#30011=CYLINDRICAL_SURFACE('',#33045,23.5) ;
#30012=CYLINDRICAL_SURFACE('',#33046,23.5) ;
#30013=CYLINDRICAL_SURFACE('',#33047,23.5) ;
#30014=CYLINDRICAL_SURFACE('',#33048,3.) ;
#30015=CYLINDRICAL_SURFACE('',#33049,3.) ;
#30016=CYLINDRICAL_SURFACE('',#33050,15.5) ;
#30017=CYLINDRICAL_SURFACE('',#33051,21.5) ;
#30018=CYLINDRICAL_SURFACE('',#33052,3.) ;
#30019=CYLINDRICAL_SURFACE('',#33053,3.) ;
#30020=CYLINDRICAL_SURFACE('',#33054,15.5) ;
#30021=CYLINDRICAL_SURFACE('',#33055,21.5) ;
#30022=CYLINDRICAL_SURFACE('',#33056,3.) ;
#30023=CYLINDRICAL_SURFACE('',#33057,3.) ;
#30024=CYLINDRICAL_SURFACE('',#33058,15.5) ;
#30025=CYLINDRICAL_SURFACE('',#33059,21.5) ;
#30749=ADVANCED_FACE('',(#2270),#29948,.F.) ;
#30750=ADVANCED_FACE('',(#2271,#1000,#1001,#1002,#1003,#1004,#1005,#1006,
#1007,#1008,#1009,#1010,#1011,#1012,#1013,#1014,#1015,#1016,#1017,#1018,
#1019),#1706,.F.) ;
#30751=ADVANCED_FACE('',(#2272),#29949,.F.) ;
#30752=ADVANCED_FACE('',(#2273),#29950,.F.) ;
#30753=ADVANCED_FACE('',(#2274,#1020,#1021),#1707,.T.) ;
#30754=ADVANCED_FACE('',(#2275),#29951,.T.) ;
#30755=ADVANCED_FACE('',(#2276),#1708,.F.) ;
#30756=ADVANCED_FACE('',(#2277,#1022,#1023),#1709,.F.) ;
#30757=ADVANCED_FACE('',(#2278),#29952,.T.) ;
#30758=ADVANCED_FACE('',(#2279),#1710,.F.) ;
#30759=ADVANCED_FACE('',(#2280,#1024,#1025),#1711,.F.) ;
#30760=ADVANCED_FACE('',(#2281),#29953,.F.) ;
#30761=ADVANCED_FACE('',(#2282),#1712,.F.) ;
#30762=ADVANCED_FACE('',(#2283),#29954,.F.) ;
#30763=ADVANCED_FACE('',(#2284),#1713,.F.) ;
#30764=ADVANCED_FACE('',(#2285),#29955,.T.) ;
#30765=ADVANCED_FACE('',(#2286),#1714,.F.) ;
#30766=ADVANCED_FACE('',(#2287,#1026,#1027,#1028,#1029,#1030,#1031,#1032,
#1033,#1034,#1035,#1036,#1037,#1038,#1039,#1040,#1041,#1042,#1043,#1044,
#1045),#1715,.T.) ;
#30767=ADVANCED_FACE('',(#2288,#1046,#1047),#1716,.F.) ;
#30768=ADVANCED_FACE('',(#2289),#1717,.T.) ;
#30769=ADVANCED_FACE('',(#2290),#29956,.F.) ;
#30770=ADVANCED_FACE('',(#2291),#29957,.F.) ;
#30771=ADVANCED_FACE('',(#2292),#29958,.F.) ;
#30772=ADVANCED_FACE('',(#2293),#29959,.F.) ;
#30773=ADVANCED_FACE('',(#2294),#29960,.F.) ;
#30774=ADVANCED_FACE('',(#2295),#903,.T.) ;
#30775=ADVANCED_FACE('',(#2296),#29961,.F.) ;
#30776=ADVANCED_FACE('',(#2297),#29962,.F.) ;
#30777=ADVANCED_FACE('',(#2298),#904,.T.) ;
#30778=ADVANCED_FACE('',(#2299),#29963,.F.) ;
#30779=ADVANCED_FACE('',(#2300),#29964,.F.) ;
#30780=ADVANCED_FACE('',(#2301),#29965,.F.) ;
#30781=ADVANCED_FACE('',(#2302),#29966,.T.) ;
#30782=ADVANCED_FACE('',(#2303),#1718,.F.) ;
#30783=ADVANCED_FACE('',(#2304),#29967,.T.) ;
#30784=ADVANCED_FACE('',(#2305),#1719,.F.) ;
#30785=ADVANCED_FACE('',(#2306),#29968,.T.) ;
#30786=ADVANCED_FACE('',(#2307),#29969,.T.) ;
#30787=ADVANCED_FACE('',(#2308),#1720,.F.) ;
#30788=ADVANCED_FACE('',(#2309),#1721,.F.) ;
#30789=ADVANCED_FACE('',(#2310),#29970,.T.) ;
#30790=ADVANCED_FACE('',(#2311),#1722,.F.) ;
#30791=ADVANCED_FACE('',(#2312),#29971,.T.) ;
#30792=ADVANCED_FACE('',(#2313),#1723,.F.) ;
#30793=ADVANCED_FACE('',(#2314),#29972,.T.) ;
#30794=ADVANCED_FACE('',(#2315),#1724,.F.) ;
#30795=ADVANCED_FACE('',(#2316),#29973,.F.) ;
#30796=ADVANCED_FACE('',(#2317),#1725,.F.) ;
#30797=ADVANCED_FACE('',(#2318),#29974,.T.) ;
#30798=ADVANCED_FACE('',(#2319),#29975,.T.) ;
#30799=ADVANCED_FACE('',(#2320),#1726,.F.) ;
#30800=ADVANCED_FACE('',(#2321),#29976,.F.) ;
#30801=ADVANCED_FACE('',(#2322),#1727,.F.) ;
#30802=ADVANCED_FACE('',(#2323),#29977,.T.) ;
#30803=ADVANCED_FACE('',(#2324),#29978,.F.) ;
#30804=ADVANCED_FACE('',(#2325),#1728,.T.) ;
#30805=ADVANCED_FACE('',(#2326),#29979,.T.) ;
#30806=ADVANCED_FACE('',(#2327),#1729,.T.) ;
#30807=ADVANCED_FACE('',(#2328),#29980,.T.) ;
#30808=ADVANCED_FACE('',(#2329),#29981,.F.) ;
#30809=ADVANCED_FACE('',(#2330),#1730,.T.) ;
#30810=ADVANCED_FACE('',(#2331),#29982,.T.) ;
#30811=ADVANCED_FACE('',(#2332),#1731,.F.) ;
#30812=ADVANCED_FACE('',(#2333),#29983,.T.) ;
#30813=ADVANCED_FACE('',(#2334),#1732,.T.) ;
#30814=ADVANCED_FACE('',(#2335),#29984,.F.) ;
#30815=ADVANCED_FACE('',(#2336),#1733,.F.) ;
#30816=ADVANCED_FACE('',(#2337),#1734,.F.) ;
#30817=ADVANCED_FACE('',(#2338),#1735,.F.) ;
#30818=ADVANCED_FACE('',(#2339),#29985,.F.) ;
#30819=ADVANCED_FACE('',(#2340),#29986,.F.) ;
#30820=ADVANCED_FACE('',(#2341),#1736,.F.) ;
#30821=ADVANCED_FACE('',(#2342),#29987,.F.) ;
#30822=ADVANCED_FACE('',(#2343),#29988,.F.) ;
#30823=ADVANCED_FACE('',(#2344),#29989,.F.) ;
#30824=ADVANCED_FACE('',(#2345),#29990,.T.) ;
#30825=ADVANCED_FACE('',(#2346),#29991,.F.) ;
#30826=ADVANCED_FACE('',(#2347),#29992,.T.) ;
#30827=ADVANCED_FACE('',(#2348),#862,.F.) ;
#30828=ADVANCED_FACE('',(#2349),#863,.F.) ;
#30829=ADVANCED_FACE('',(#2350),#1737,.F.) ;
#30830=ADVANCED_FACE('',(#2351),#1738,.F.) ;
#30831=ADVANCED_FACE('',(#2352),#29993,.F.) ;
#30832=ADVANCED_FACE('',(#2353),#29994,.F.) ;
#30833=ADVANCED_FACE('',(#2354),#29995,.F.) ;
#30834=ADVANCED_FACE('',(#2355),#29996,.F.) ;
#30835=ADVANCED_FACE('',(#2356),#29997,.F.) ;
#30836=ADVANCED_FACE('',(#2357),#1739,.F.) ;
#30837=ADVANCED_FACE('',(#2358),#29998,.F.) ;
#30838=ADVANCED_FACE('',(#2359),#1740,.F.) ;
#30839=ADVANCED_FACE('',(#2360),#29999,.F.) ;
#30840=ADVANCED_FACE('',(#2361),#1741,.F.) ;
#30841=ADVANCED_FACE('',(#2362),#30000,.F.) ;
#30842=ADVANCED_FACE('',(#2363),#1742,.F.) ;
#30843=ADVANCED_FACE('',(#2364),#30001,.F.) ;
#30844=ADVANCED_FACE('',(#2365),#1743,.F.) ;
#30845=ADVANCED_FACE('',(#2366),#30002,.F.) ;
#30846=ADVANCED_FACE('',(#2367),#1744,.F.) ;
#30847=ADVANCED_FACE('',(#2368),#30003,.F.) ;
#30848=ADVANCED_FACE('',(#2369),#1745,.F.) ;
#30849=ADVANCED_FACE('',(#2370),#30004,.F.) ;
#30850=ADVANCED_FACE('',(#2371),#1746,.F.) ;
#30851=ADVANCED_FACE('',(#2372),#30005,.F.) ;
#30852=ADVANCED_FACE('',(#2373),#1747,.F.) ;
#30853=ADVANCED_FACE('',(#2374),#30006,.F.) ;
#30854=ADVANCED_FACE('',(#2375),#1748,.F.) ;
#30855=ADVANCED_FACE('',(#2376),#30007,.F.) ;
#30856=ADVANCED_FACE('',(#2377),#1749,.F.) ;
#30857=ADVANCED_FACE('',(#2378),#30008,.F.) ;
#30858=ADVANCED_FACE('',(#2379),#1750,.F.) ;
#30859=ADVANCED_FACE('',(#2380),#30009,.T.) ;
#30860=ADVANCED_FACE('',(#2381),#1751,.F.) ;
#30861=ADVANCED_FACE('',(#2382),#30010,.F.) ;
#30862=ADVANCED_FACE('',(#2383),#30011,.T.) ;
#30863=ADVANCED_FACE('',(#2384),#30012,.T.) ;
#30864=ADVANCED_FACE('',(#2385),#30013,.T.) ;
#30865=ADVANCED_FACE('',(#2386),#30014,.F.) ;
#30866=ADVANCED_FACE('',(#2387),#30015,.F.) ;
#30867=ADVANCED_FACE('',(#2388),#30016,.T.) ;
#30868=ADVANCED_FACE('',(#2389),#30017,.F.) ;
#30869=ADVANCED_FACE('',(#2390),#30018,.F.) ;
#30870=ADVANCED_FACE('',(#2391),#30019,.F.) ;
#30871=ADVANCED_FACE('',(#2392),#30020,.T.) ;
#30872=ADVANCED_FACE('',(#2393),#30021,.F.) ;
#30873=ADVANCED_FACE('',(#2394),#30022,.F.) ;
#30874=ADVANCED_FACE('',(#2395),#30023,.F.) ;
#30875=ADVANCED_FACE('',(#2396),#30024,.T.) ;
#30876=ADVANCED_FACE('',(#2397),#30025,.F.) ;
#32637=CLOSED_SHELL('',(#30749,#30750,#30751,#30752,#30753,#30754,#30755,
#30756,#30757,#30758,#30759,#30760,#30761,#30762,#30763,#30764,#30765,#30766,
#30767,#30768,#30769,#30770,#30771,#30772,#30773,#30774,#30775,#30776,#30777,
#30778,#30779,#30780,#30781,#30782,#30783,#30784,#30785,#30786,#30787,#30788,
#30789,#30790,#30791,#30792,#30793,#30794,#30795,#30796,#30797,#30798,#30799,
#30800,#30801,#30802,#30803,#30804,#30805,#30806,#30807,#30808,#30809,#30810,
#30811,#30812,#30813,#30814,#30815,#30816,#30817,#30818,#30819,#30820,#30821,
#30822,#30823,#30824,#30825,#30826,#30827,#30828,#30829,#30830,#30831,#30832,
#30833,#30834,#30835,#30836,#30837,#30838,#30839,#30840,#30841,#30842,#30843,
#30844,#30845,#30846,#30847,#30848,#30849,#30850,#30851,#30852,#30853,#30854,
#30855,#30856,#30857,#30858,#30859,#30860,#30861,#30862,#30863,#30864,#30865,
#30866,#30867,#30868,#30869,#30870,#30871,#30872,#30873,#30874,#30875,#30876)) ;
#32773=AXIS2_PLACEMENT_3D('',#46348,#36527,#36528) ;
#32774=AXIS2_PLACEMENT_3D('',#46349,#36529,#36530) ;
#32775=AXIS2_PLACEMENT_3D('',#46352,#36531,#36532) ;
#32776=AXIS2_PLACEMENT_3D('',#46356,#36534,#36535) ;
#32777=AXIS2_PLACEMENT_3D('',#46358,#36537,#36538) ;
#32778=AXIS2_PLACEMENT_3D('',#46370,#36544,#36545) ;
#32779=AXIS2_PLACEMENT_3D('',#46380,#36546,#36547) ;
#32780=AXIS2_PLACEMENT_3D('',#46381,#36548,#36549) ;
#32781=AXIS2_PLACEMENT_3D('',#46392,#36550,#36551) ;
#32782=AXIS2_PLACEMENT_3D('',#46394,#36552,#36553) ;
#32783=AXIS2_PLACEMENT_3D('',#46395,#36554,#36555) ;
#32784=AXIS2_PLACEMENT_3D('',#46398,#36556,#36557) ;
#32785=AXIS2_PLACEMENT_3D('',#46400,#36558,#36559) ;
#32786=AXIS2_PLACEMENT_3D('',#46402,#36560,#36561) ;
#32787=AXIS2_PLACEMENT_3D('',#46403,#36562,#36563) ;
#32788=AXIS2_PLACEMENT_3D('',#46406,#36564,#36565) ;
#32789=AXIS2_PLACEMENT_3D('',#46408,#36566,#36567) ;
#32790=AXIS2_PLACEMENT_3D('',#46410,#36568,#36569) ;
#32791=AXIS2_PLACEMENT_3D('',#46411,#36570,#36571) ;
#32792=AXIS2_PLACEMENT_3D('',#46416,#36573,#36574) ;
#32793=AXIS2_PLACEMENT_3D('',#46419,#36576,#36577) ;
#32794=AXIS2_PLACEMENT_3D('',#46424,#36579,#36580) ;
#32795=AXIS2_PLACEMENT_3D('',#46427,#36582,#36583) ;
#32796=AXIS2_PLACEMENT_3D('',#46432,#36585,#36586) ;
#32797=AXIS2_PLACEMENT_3D('',#46435,#36588,#36589) ;
#32798=AXIS2_PLACEMENT_3D('',#46440,#36591,#36592) ;
#32799=AXIS2_PLACEMENT_3D('',#46443,#36594,#36595) ;
#32800=AXIS2_PLACEMENT_3D('',#46448,#36597,#36598) ;
#32801=AXIS2_PLACEMENT_3D('',#46451,#36600,#36601) ;
#32802=AXIS2_PLACEMENT_3D('',#46456,#36603,#36604) ;
#32803=AXIS2_PLACEMENT_3D('',#46459,#36606,#36607) ;
#32804=AXIS2_PLACEMENT_3D('',#46461,#36608,#36609) ;
#32805=AXIS2_PLACEMENT_3D('',#46463,#36610,#36611) ;
#32806=AXIS2_PLACEMENT_3D('',#46465,#36612,#36613) ;
#32807=AXIS2_PLACEMENT_3D('',#46467,#36614,#36615) ;
#32808=AXIS2_PLACEMENT_3D('',#46469,#36616,#36617) ;
#32809=AXIS2_PLACEMENT_3D('',#46471,#36618,#36619) ;
#32810=AXIS2_PLACEMENT_3D('',#46474,#36620,#36621) ;
#32811=AXIS2_PLACEMENT_3D('',#46476,#36622,#36623) ;
#32812=AXIS2_PLACEMENT_3D('',#46478,#36624,#36625) ;
#32813=AXIS2_PLACEMENT_3D('',#46479,#36626,#36627) ;
#32814=AXIS2_PLACEMENT_3D('',#46482,#36628,#36629) ;
#32815=AXIS2_PLACEMENT_3D('',#46484,#36630,#36631) ;
#32816=AXIS2_PLACEMENT_3D('',#46486,#36632,#36633) ;
#32817=AXIS2_PLACEMENT_3D('',#46487,#36634,#36635) ;
#32818=AXIS2_PLACEMENT_3D('',#46490,#36636,#36637) ;
#32819=AXIS2_PLACEMENT_3D('',#46492,#36638,#36639) ;
#32820=AXIS2_PLACEMENT_3D('',#46494,#36640,#36641) ;
#32821=AXIS2_PLACEMENT_3D('',#46495,#36642,#36643) ;
#32822=AXIS2_PLACEMENT_3D('',#46498,#36644,#36645) ;
#32823=AXIS2_PLACEMENT_3D('',#46500,#36646,#36647) ;
#32824=AXIS2_PLACEMENT_3D('',#46502,#36648,#36649) ;
#32825=AXIS2_PLACEMENT_3D('',#46503,#36650,#36651) ;
#32826=AXIS2_PLACEMENT_3D('',#46504,#36652,#36653) ;
#32827=AXIS2_PLACEMENT_3D('',#46506,#36654,#36655) ;
#32828=AXIS2_PLACEMENT_3D('',#46508,#36656,#36657) ;
#32829=AXIS2_PLACEMENT_3D('',#46510,#36659,#36660) ;
#32830=AXIS2_PLACEMENT_3D('',#46512,#36661,#36662) ;
#32831=AXIS2_PLACEMENT_3D('',#46515,#36664,#36665) ;
#32832=AXIS2_PLACEMENT_3D('',#46516,#36666,#36667) ;
#32833=AXIS2_PLACEMENT_3D('',#46520,#36669,#36670) ;
#32834=AXIS2_PLACEMENT_3D('',#46524,#36672,#36673) ;
#32835=AXIS2_PLACEMENT_3D('',#46528,#36675,#36676) ;
#32836=AXIS2_PLACEMENT_3D('',#46532,#36678,#36679) ;
#32837=AXIS2_PLACEMENT_3D('',#46536,#36681,#36682) ;
#32838=AXIS2_PLACEMENT_3D('',#46540,#36684,#36685) ;
#32839=AXIS2_PLACEMENT_3D('',#46544,#36687,#36688) ;
#32840=AXIS2_PLACEMENT_3D('',#46548,#36690,#36691) ;
#32841=AXIS2_PLACEMENT_3D('',#46551,#36693,#36694) ;
#32842=AXIS2_PLACEMENT_3D('',#46553,#36695,#36696) ;
#32843=AXIS2_PLACEMENT_3D('',#46554,#36697,#36698) ;
#32844=AXIS2_PLACEMENT_3D('',#46557,#36699,#36700) ;
#32845=AXIS2_PLACEMENT_3D('',#46561,#36702,#36703) ;
#32846=AXIS2_PLACEMENT_3D('',#46563,#36705,#36706) ;
#32847=AXIS2_PLACEMENT_3D('',#46572,#36712,#36713) ;
#32848=AXIS2_PLACEMENT_3D('',#46576,#36715,#36716) ;
#32849=AXIS2_PLACEMENT_3D('',#46580,#36718,#36719) ;
#32850=AXIS2_PLACEMENT_3D('',#46584,#36721,#36722) ;
#32851=AXIS2_PLACEMENT_3D('',#46588,#36724,#36725) ;
#32852=AXIS2_PLACEMENT_3D('',#46592,#36727,#36728) ;
#32853=AXIS2_PLACEMENT_3D('',#46596,#36730,#36731) ;
#32854=AXIS2_PLACEMENT_3D('',#46600,#36733,#36734) ;
#32855=AXIS2_PLACEMENT_3D('',#46603,#36736,#36737) ;
#32856=AXIS2_PLACEMENT_3D('',#46605,#36738,#36739) ;
#32857=AXIS2_PLACEMENT_3D('',#46607,#36740,#36741) ;
#32858=AXIS2_PLACEMENT_3D('',#46608,#36742,#36743) ;
#32859=AXIS2_PLACEMENT_3D('',#46611,#36744,#36745) ;
#32860=AXIS2_PLACEMENT_3D('',#46615,#36747,#36748) ;
#32861=AXIS2_PLACEMENT_3D('',#46617,#36750,#36751) ;
#32862=AXIS2_PLACEMENT_3D('',#46624,#36756,#36757) ;
#32863=AXIS2_PLACEMENT_3D('',#46628,#36759,#36760) ;
#32864=AXIS2_PLACEMENT_3D('',#46632,#36762,#36763) ;
#32865=AXIS2_PLACEMENT_3D('',#46636,#36765,#36766) ;
#32866=AXIS2_PLACEMENT_3D('',#46640,#36768,#36769) ;
#32867=AXIS2_PLACEMENT_3D('',#46644,#36771,#36772) ;
#32868=AXIS2_PLACEMENT_3D('',#46648,#36774,#36775) ;
#32869=AXIS2_PLACEMENT_3D('',#46652,#36777,#36778) ;
#32870=AXIS2_PLACEMENT_3D('',#46655,#36780,#36781) ;
#32871=AXIS2_PLACEMENT_3D('',#46657,#36782,#36783) ;
#32872=AXIS2_PLACEMENT_3D('',#46659,#36784,#36785) ;
#32873=AXIS2_PLACEMENT_3D('',#46660,#36786,#36787) ;
#32874=AXIS2_PLACEMENT_3D('',#46664,#36789,#36790) ;
#32875=AXIS2_PLACEMENT_3D('',#46666,#36792,#36793) ;
#32876=AXIS2_PLACEMENT_3D('',#46670,#36796,#36797) ;
#32877=AXIS2_PLACEMENT_3D('',#46673,#36800,#36801) ;
#32878=AXIS2_PLACEMENT_3D('',#46675,#36803,#36804) ;
#32879=AXIS2_PLACEMENT_3D('',#46678,#36805,#36806) ;
#32880=AXIS2_PLACEMENT_3D('',#46682,#36808,#36809) ;
#32881=AXIS2_PLACEMENT_3D('',#46684,#36811,#36812) ;
#32882=AXIS2_PLACEMENT_3D('',#46691,#36817,#36818) ;
#32883=AXIS2_PLACEMENT_3D('',#46704,#36825,#36826) ;
#32884=AXIS2_PLACEMENT_3D('',#46706,#36827,#36828) ;
#32885=AXIS2_PLACEMENT_3D('',#46708,#36829,#36830) ;
#32886=AXIS2_PLACEMENT_3D('',#46709,#36831,#36832) ;
#32887=AXIS2_PLACEMENT_3D('',#46711,#36833,#36834) ;
#32888=AXIS2_PLACEMENT_3D('',#46713,#36835,#36836) ;
#32889=AXIS2_PLACEMENT_3D('',#46716,#36837,#36838) ;
#32890=AXIS2_PLACEMENT_3D('',#46720,#36840,#36841) ;
#32891=AXIS2_PLACEMENT_3D('',#46724,#36843,#36844) ;
#32892=AXIS2_PLACEMENT_3D('',#46728,#36846,#36847) ;
#32893=AXIS2_PLACEMENT_3D('',#46732,#36849,#36850) ;
#32894=AXIS2_PLACEMENT_3D('',#46736,#36852,#36853) ;
#32895=AXIS2_PLACEMENT_3D('',#46740,#36855,#36856) ;
#32896=AXIS2_PLACEMENT_3D('',#46744,#36858,#36859) ;
#32897=AXIS2_PLACEMENT_3D('',#46748,#36861,#36862) ;
#32898=AXIS2_PLACEMENT_3D('',#46752,#36864,#36865) ;
#32899=AXIS2_PLACEMENT_3D('',#46756,#36867,#36868) ;
#32900=AXIS2_PLACEMENT_3D('',#46760,#36870,#36871) ;
#32901=AXIS2_PLACEMENT_3D('',#46763,#36873,#36874) ;
#32902=AXIS2_PLACEMENT_3D('',#46765,#36875,#36876) ;
#32903=AXIS2_PLACEMENT_3D('',#46767,#36877,#36878) ;
#32904=AXIS2_PLACEMENT_3D('',#46769,#36879,#36880) ;
#32905=AXIS2_PLACEMENT_3D('',#46772,#36881,#36882) ;
#32906=AXIS2_PLACEMENT_3D('',#46774,#36883,#36884) ;
#32907=AXIS2_PLACEMENT_3D('',#46776,#36885,#36886) ;
#32908=AXIS2_PLACEMENT_3D('',#46777,#36887,#36888) ;
#32909=AXIS2_PLACEMENT_3D('',#46780,#36889,#36890) ;
#32910=AXIS2_PLACEMENT_3D('',#46782,#36891,#36892) ;
#32911=AXIS2_PLACEMENT_3D('',#46784,#36893,#36894) ;
#32912=AXIS2_PLACEMENT_3D('',#46785,#36895,#36896) ;
#32913=AXIS2_PLACEMENT_3D('',#46788,#36897,#36898) ;
#32914=AXIS2_PLACEMENT_3D('',#46790,#36899,#36900) ;
#32915=AXIS2_PLACEMENT_3D('',#46792,#36901,#36902) ;
#32916=AXIS2_PLACEMENT_3D('',#46793,#36903,#36904) ;
#32917=AXIS2_PLACEMENT_3D('',#46796,#36905,#36906) ;
#32918=AXIS2_PLACEMENT_3D('',#46798,#36907,#36908) ;
#32919=AXIS2_PLACEMENT_3D('',#46800,#36909,#36910) ;
#32920=AXIS2_PLACEMENT_3D('',#46801,#36911,#36912) ;
#32921=AXIS2_PLACEMENT_3D('',#46804,#36913,#36914) ;
#32922=AXIS2_PLACEMENT_3D('',#46806,#36915,#36916) ;
#32923=AXIS2_PLACEMENT_3D('',#46808,#36917,#36918) ;
#32924=AXIS2_PLACEMENT_3D('',#46809,#36919,#36920) ;
#32925=AXIS2_PLACEMENT_3D('',#46812,#36921,#36922) ;
#32926=AXIS2_PLACEMENT_3D('',#46814,#36923,#36924) ;
#32927=AXIS2_PLACEMENT_3D('',#46816,#36925,#36926) ;
#32928=AXIS2_PLACEMENT_3D('',#46826,#36927,#36928) ;
#32929=AXIS2_PLACEMENT_3D('',#46828,#36929,#36930) ;
#32930=AXIS2_PLACEMENT_3D('',#46830,#36931,#36932) ;
#32931=AXIS2_PLACEMENT_3D('',#46838,#36933,#36934) ;
#32932=AXIS2_PLACEMENT_3D('',#46840,#36935,#36936) ;
#32933=AXIS2_PLACEMENT_3D('',#46844,#36938,#36939) ;
#32934=AXIS2_PLACEMENT_3D('',#46848,#36941,#36942) ;
#32935=AXIS2_PLACEMENT_3D('',#46852,#36944,#36945) ;
#32936=AXIS2_PLACEMENT_3D('',#46856,#36947,#36948) ;
#32937=AXIS2_PLACEMENT_3D('',#46860,#36950,#36951) ;
#32938=AXIS2_PLACEMENT_3D('',#46863,#36953,#36954) ;
#32939=AXIS2_PLACEMENT_3D('',#46866,#36956,#36957) ;
#32940=AXIS2_PLACEMENT_3D('',#46868,#36958,#36959) ;
#32941=AXIS2_PLACEMENT_3D('',#46869,#36960,#36961) ;
#32942=AXIS2_PLACEMENT_3D('',#46873,#36963,#36964) ;
#32943=AXIS2_PLACEMENT_3D('',#46876,#36966,#36967) ;
#32944=AXIS2_PLACEMENT_3D('',#46877,#36968,#36969) ;
#32945=AXIS2_PLACEMENT_3D('',#46880,#36972,#36973) ;
#32946=AXIS2_PLACEMENT_3D('',#46882,#36975,#36976) ;
#32947=AXIS2_PLACEMENT_3D('',#46885,#36979,#36980) ;
#32948=AXIS2_PLACEMENT_3D('',#46887,#36982,#36983) ;
#32949=AXIS2_PLACEMENT_3D('',#46919,#36987,#36988) ;
#32950=AXIS2_PLACEMENT_3D('',#46921,#36990,#36991) ;
#32951=AXIS2_PLACEMENT_3D('',#46953,#36995,#36996) ;
#32952=AXIS2_PLACEMENT_3D('',#46955,#36998,#36999) ;
#32953=AXIS2_PLACEMENT_3D('',#46957,#37001,#37002) ;
#32954=AXIS2_PLACEMENT_3D('',#46959,#37004,#37005) ;
#32955=AXIS2_PLACEMENT_3D('',#46962,#37007,#37008) ;
#32956=AXIS2_PLACEMENT_3D('',#46963,#37009,#37010) ;
#32957=AXIS2_PLACEMENT_3D('',#46967,#37013,#37014) ;
#32958=AXIS2_PLACEMENT_3D('',#46970,#37016,#37017) ;
#32959=AXIS2_PLACEMENT_3D('',#46971,#37018,#37019) ;
#32960=AXIS2_PLACEMENT_3D('',#46974,#37022,#37023) ;
#32961=AXIS2_PLACEMENT_3D('',#46975,#37024,#37025) ;
#32962=AXIS2_PLACEMENT_3D('',#46978,#37026,#37027) ;
#32963=AXIS2_PLACEMENT_3D('',#46982,#37029,#37030) ;
#32964=AXIS2_PLACEMENT_3D('',#46984,#37032,#37033) ;
#32965=AXIS2_PLACEMENT_3D('',#46990,#37037,#37038) ;
#32966=AXIS2_PLACEMENT_3D('',#46997,#37042,#37043) ;
#32967=AXIS2_PLACEMENT_3D('',#46998,#37044,#37045) ;
#32968=AXIS2_PLACEMENT_3D('',#47000,#37046,#37047) ;
#32969=AXIS2_PLACEMENT_3D('',#47002,#37049,#37050) ;
#32970=AXIS2_PLACEMENT_3D('',#47004,#37051,#37052) ;
#32971=AXIS2_PLACEMENT_3D('',#47006,#37054,#37055) ;
#32972=AXIS2_PLACEMENT_3D('',#47008,#37057,#37058) ;
#32973=AXIS2_PLACEMENT_3D('',#47010,#37060,#37061) ;
#32974=AXIS2_PLACEMENT_3D('',#47011,#37062,#37063) ;
#32975=AXIS2_PLACEMENT_3D('',#47014,#37066,#37067) ;
#32976=AXIS2_PLACEMENT_3D('',#47016,#37069,#37070) ;
#32977=AXIS2_PLACEMENT_3D('',#47019,#37073,#37074) ;
#32978=AXIS2_PLACEMENT_3D('',#47021,#37076,#37077) ;
#32979=AXIS2_PLACEMENT_3D('',#47022,#37078,#37079) ;
#32980=AXIS2_PLACEMENT_3D('',#47025,#37082,#37083) ;
#32981=AXIS2_PLACEMENT_3D('',#47027,#37085,#37086) ;
#32982=AXIS2_PLACEMENT_3D('',#47030,#37089,#37090) ;
#32983=AXIS2_PLACEMENT_3D('',#47031,#37091,#37092) ;
#32984=AXIS2_PLACEMENT_3D('',#47033,#37094,#37095) ;
#32985=AXIS2_PLACEMENT_3D('',#47036,#37098,#37099) ;
#32986=AXIS2_PLACEMENT_3D('',#47038,#37101,#37102) ;
#32987=AXIS2_PLACEMENT_3D('',#47040,#37104,#37105) ;
#32988=AXIS2_PLACEMENT_3D('',#47042,#37107,#37108) ;
#32989=AXIS2_PLACEMENT_3D('',#47043,#37109,#37110) ;
#32990=AXIS2_PLACEMENT_3D('',#47046,#37113,#37114) ;
#32991=AXIS2_PLACEMENT_3D('',#47048,#37116,#37117) ;
#32992=AXIS2_PLACEMENT_3D('',#47050,#37119,#37120) ;
#32993=AXIS2_PLACEMENT_3D('',#47052,#37122,#37123) ;
#32994=AXIS2_PLACEMENT_3D('',#47054,#37125,#37126) ;
#32995=AXIS2_PLACEMENT_3D('',#47055,#37127,#37128) ;
#32996=AXIS2_PLACEMENT_3D('',#47056,#37129,#37130) ;
#32997=AXIS2_PLACEMENT_3D('',#47057,#37131,#37132) ;
#32998=AXIS2_PLACEMENT_3D('',#47060,#37134,#37135) ;
#32999=AXIS2_PLACEMENT_3D('',#47061,#37136,#37137) ;
#33000=AXIS2_PLACEMENT_3D('',#47062,#37138,#37139) ;
#33001=AXIS2_PLACEMENT_3D('',#47063,#37140,#37141) ;
#33002=AXIS2_PLACEMENT_3D('',#47065,#37143,#37144) ;
#33003=AXIS2_PLACEMENT_3D('',#47067,#37146,#37147) ;
#33004=AXIS2_PLACEMENT_3D('',#47068,#37148,#37149) ;
#33005=AXIS2_PLACEMENT_3D('',#47070,#37151,#37152) ;
#33006=AXIS2_PLACEMENT_3D('',#47073,#37155,#37156) ;
#33007=AXIS2_PLACEMENT_3D('',#47076,#37159,#37160) ;
#33008=AXIS2_PLACEMENT_3D('',#47077,#37161,#37162) ;
#33009=AXIS2_PLACEMENT_3D('',#47078,#37163,#37164) ;
#33010=AXIS2_PLACEMENT_3D('',#47079,#37165,#37166) ;
#33011=AXIS2_PLACEMENT_3D('',#47081,#37168,#37169) ;
#33012=AXIS2_PLACEMENT_3D('',#47083,#37171,#37172) ;
#33013=AXIS2_PLACEMENT_3D('',#47084,#37173,#37174) ;
#33014=AXIS2_PLACEMENT_3D('',#47085,#37175,#37176) ;
#33015=AXIS2_PLACEMENT_3D('',#47087,#37178,#37179) ;
#33016=AXIS2_PLACEMENT_3D('',#47089,#37181,#37182) ;
#33017=AXIS2_PLACEMENT_3D('',#47091,#37184,#37185) ;
#33018=AXIS2_PLACEMENT_3D('',#47093,#37187,#37188) ;
#33019=AXIS2_PLACEMENT_3D('',#47096,#37191,#37192) ;
#33020=AXIS2_PLACEMENT_3D('',#47098,#37194,#37195) ;
#33021=AXIS2_PLACEMENT_3D('',#47100,#37197,#37198) ;
#33022=AXIS2_PLACEMENT_3D('',#47101,#37199,#37200) ;
#33023=AXIS2_PLACEMENT_3D('',#47104,#37203,#37204) ;
#33024=AXIS2_PLACEMENT_3D('',#47106,#37206,#37207) ;
#33025=AXIS2_PLACEMENT_3D('',#47108,#37209,#37210) ;
#33026=AXIS2_PLACEMENT_3D('',#47109,#37211,#37212) ;
#33027=AXIS2_PLACEMENT_3D('',#47112,#37215,#37216) ;
#33028=AXIS2_PLACEMENT_3D('',#47114,#37218,#37219) ;
#33029=AXIS2_PLACEMENT_3D('',#47116,#37221,#37222) ;
#33030=AXIS2_PLACEMENT_3D('',#47117,#37223,#37224) ;
#33031=AXIS2_PLACEMENT_3D('',#47120,#37227,#37228) ;
#33032=AXIS2_PLACEMENT_3D('',#47122,#37230,#37231) ;
#33033=AXIS2_PLACEMENT_3D('',#47124,#37233,#37234) ;
#33034=AXIS2_PLACEMENT_3D('',#47125,#37235,#37236) ;
#33035=AXIS2_PLACEMENT_3D('',#47128,#37239,#37240) ;
#33036=AXIS2_PLACEMENT_3D('',#47130,#37242,#37243) ;
#33037=AXIS2_PLACEMENT_3D('',#47132,#37245,#37246) ;
#33038=AXIS2_PLACEMENT_3D('',#47133,#37247,#37248) ;
#33039=AXIS2_PLACEMENT_3D('',#47136,#37251,#37252) ;
#33040=AXIS2_PLACEMENT_3D('',#47138,#37254,#37255) ;
#33041=AXIS2_PLACEMENT_3D('',#47140,#37257,#37258) ;
#33042=AXIS2_PLACEMENT_3D('',#47141,#37259,#37260) ;
#33043=AXIS2_PLACEMENT_3D('',#47143,#37262,#37263) ;
#33044=AXIS2_PLACEMENT_3D('',#47144,#37264,#37265) ;
#33045=AXIS2_PLACEMENT_3D('',#47146,#37267,#37268) ;
#33046=AXIS2_PLACEMENT_3D('',#47147,#37269,#37270) ;
#33047=AXIS2_PLACEMENT_3D('',#47148,#37271,#37272) ;
#33048=AXIS2_PLACEMENT_3D('',#47149,#37273,#37274) ;
#33049=AXIS2_PLACEMENT_3D('',#47152,#37277,#37278) ;
#33050=AXIS2_PLACEMENT_3D('',#47155,#37281,#37282) ;
#33051=AXIS2_PLACEMENT_3D('',#47156,#37283,#37284) ;
#33052=AXIS2_PLACEMENT_3D('',#47157,#37285,#37286) ;
#33053=AXIS2_PLACEMENT_3D('',#47160,#37289,#37290) ;
#33054=AXIS2_PLACEMENT_3D('',#47163,#37293,#37294) ;
#33055=AXIS2_PLACEMENT_3D('',#47164,#37295,#37296) ;
#33056=AXIS2_PLACEMENT_3D('',#47165,#37297,#37298) ;
#33057=AXIS2_PLACEMENT_3D('',#47168,#37301,#37302) ;
#33058=AXIS2_PLACEMENT_3D('',#47171,#37305,#37306) ;
#33059=AXIS2_PLACEMENT_3D('',#47172,#37307,#37308) ;
#36527=DIRECTION('axis',(0.,0.,1.)) ;
#36528=DIRECTION('refdir',(1.,0.,0.)) ;
#36529=DIRECTION('center_axis',(-1.,1.75658099177411E-13,4.54195640846217E-14)) ;
#36530=DIRECTION('ref_axis',(1.56325514861445E-13,0.707106781186434,0.707106781186661)) ;
#36531=DIRECTION('center_axis',(1.,-1.75658099177411E-13,-4.54195640846217E-14)) ;
#36532=DIRECTION('ref_axis',(1.56325514861445E-13,0.707106781186434,0.707106781186661)) ;
#36533=DIRECTION('',(-1.,1.75658099177411E-13,4.54195640846217E-14)) ;
#36534=DIRECTION('center_axis',(-1.,1.75658099177411E-13,4.54195640846217E-14)) ;
#36535=DIRECTION('ref_axis',(1.56325514861445E-13,0.707106781186434,0.707106781186661)) ;
#36536=DIRECTION('',(1.,-1.75658099177411E-13,-4.54195640846217E-14)) ;
#36537=DIRECTION('center_axis',(4.54195640846217E-14,-1.66321791214601E-16,
1.)) ;
#36538=DIRECTION('ref_axis',(1.,-1.75658099177411E-13,-4.54195640846217E-14)) ;
#36539=DIRECTION('',(1.75658099177411E-13,1.,1.66321791206623E-16)) ;
#36540=DIRECTION('',(1.,-1.75658099177411E-13,-4.54195640846217E-14)) ;
#36541=DIRECTION('',(1.75658099177411E-13,1.,1.66321791206623E-16)) ;
#36542=DIRECTION('',(-1.75658099177411E-13,-1.,-1.66321791206623E-16)) ;
#36543=DIRECTION('',(1.75658099177411E-13,1.,1.66321791206623E-16)) ;
#36544=DIRECTION('center_axis',(4.54195640846217E-14,-1.66321791214601E-16,
1.)) ;
#36545=DIRECTION('ref_axis',(-0.866025403784527,-0.499999999999848,3.92513354304944E-14)) ;
#36546=DIRECTION('center_axis',(4.54195640846217E-14,-1.66321791214601E-16,
1.)) ;
#36547=DIRECTION('ref_axis',(-1.,5.55236256206829E-46,4.54195640846217E-14)) ;
#36548=DIRECTION('center_axis',(-4.54195640846217E-14,1.66321791214601E-16,
-1.)) ;
#36549=DIRECTION('ref_axis',(0.156304737392435,0.987708878702972,-6.93501552682122E-15)) ;
#36550=DIRECTION('center_axis',(4.54195640846217E-14,-1.66321791214601E-16,
1.)) ;
#36551=DIRECTION('ref_axis',(-1.,5.55236256206829E-46,4.54195640846217E-14)) ;
#36552=DIRECTION('center_axis',(-4.54195640846217E-14,1.66321791214601E-16,
-1.)) ;
#36553=DIRECTION('ref_axis',(0.987708878702962,-0.1563047373925,-4.48873035970975E-14)) ;
#36554=DIRECTION('center_axis',(4.54195640846217E-14,-1.66321791214601E-16,
1.)) ;
#36555=DIRECTION('ref_axis',(-0.499999999999848,0.866025403784526,2.28538209386987E-14)) ;
#36556=DIRECTION('center_axis',(-4.54195640846217E-14,1.66321791214601E-16,
-1.)) ;
#36557=DIRECTION('ref_axis',(0.987707474797848,0.156313608583704,-4.48352445890699E-14)) ;
#36558=DIRECTION('center_axis',(4.54195640846217E-14,-1.66321791214601E-16,
1.)) ;
#36559=DIRECTION('ref_axis',(-1.,5.55236256206829E-46,4.54195640846217E-14)) ;
#36560=DIRECTION('center_axis',(-4.54195640846217E-14,1.66321791214601E-16,
-1.)) ;
#36561=DIRECTION('ref_axis',(-0.156304737392422,-0.987708878702974,6.93501552682063E-15)) ;
#36562=DIRECTION('center_axis',(4.54195640846217E-14,-1.66321791214601E-16,
1.)) ;
#36563=DIRECTION('ref_axis',(0.866025403784527,0.499999999999848,-3.92513354304944E-14)) ;
#36564=DIRECTION('center_axis',(4.54195640846217E-14,-1.66321791214601E-16,
1.)) ;
#36565=DIRECTION('ref_axis',(-1.,1.75719331517368E-13,4.54195640846217E-14)) ;
#36566=DIRECTION('center_axis',(4.54195640846217E-14,-1.66321791214601E-16,
1.)) ;
#36567=DIRECTION('ref_axis',(-0.965925826289023,0.25881904510269,4.39149772153074E-14)) ;
#36568=DIRECTION('center_axis',(4.54195640846217E-14,-1.66321791214601E-16,
1.)) ;
#36569=DIRECTION('ref_axis',(-1.,1.75719331517368E-13,4.54195640846217E-14)) ;
#36570=DIRECTION('center_axis',(4.54195640846217E-14,-1.66321791214601E-16,
1.)) ;
#36571=DIRECTION('ref_axis',(-0.965925826289114,-0.258819045102351,4.38288827209477E-14)) ;
#36572=DIRECTION('',(-1.75658099177411E-13,-1.,-1.66321791206623E-16)) ;
#36573=DIRECTION('center_axis',(4.54195640846217E-14,-1.66321791214601E-16,
1.)) ;
#36574=DIRECTION('ref_axis',(1.75658099177411E-13,1.,1.66321791206623E-16)) ;
#36575=DIRECTION('',(1.75658099177411E-13,1.,1.66321791206623E-16)) ;
#36576=DIRECTION('center_axis',(4.54195640846217E-14,-1.66321791214601E-16,
1.)) ;
#36577=DIRECTION('ref_axis',(1.75658099177411E-13,1.,1.66321791206623E-16)) ;
#36578=DIRECTION('',(-1.75658099177411E-13,-1.,-1.66321791206623E-16)) ;
#36579=DIRECTION('center_axis',(4.54195640846217E-14,-1.66321791214601E-16,
1.)) ;
#36580=DIRECTION('ref_axis',(1.75658099177411E-13,1.,1.66321791206623E-16)) ;
#36581=DIRECTION('',(1.75658099177411E-13,1.,1.66321791206623E-16)) ;
#36582=DIRECTION('center_axis',(4.54195640846217E-14,-1.66321791214601E-16,
1.)) ;
#36583=DIRECTION('ref_axis',(1.75658099177411E-13,1.,1.66321791206623E-16)) ;
#36584=DIRECTION('',(-1.75658099177411E-13,-1.,-1.66321791206623E-16)) ;
#36585=DIRECTION('center_axis',(4.54195640846217E-14,-1.66321791214601E-16,
1.)) ;
#36586=DIRECTION('ref_axis',(1.75658099177411E-13,1.,1.66321791206623E-16)) ;
#36587=DIRECTION('',(1.75658099177411E-13,1.,1.66321791206623E-16)) ;
#36588=DIRECTION('center_axis',(4.54195640846217E-14,-1.66321791214601E-16,
1.)) ;
#36589=DIRECTION('ref_axis',(1.75658099177411E-13,1.,1.66321791206623E-16)) ;
#36590=DIRECTION('',(-1.75658099177411E-13,-1.,-1.66321791206623E-16)) ;
#36591=DIRECTION('center_axis',(4.54195640846217E-14,-1.66321791214601E-16,
1.)) ;
#36592=DIRECTION('ref_axis',(1.75658099177411E-13,1.,1.66321791206623E-16)) ;
#36593=DIRECTION('',(1.75658099177411E-13,1.,1.66321791206623E-16)) ;
#36594=DIRECTION('center_axis',(4.54195640846217E-14,-1.66321791214601E-16,
1.)) ;
#36595=DIRECTION('ref_axis',(1.75658099177411E-13,1.,1.66321791206623E-16)) ;
#36596=DIRECTION('',(1.75658099177411E-13,1.,1.66321791206623E-16)) ;
#36597=DIRECTION('center_axis',(4.54195640846217E-14,-1.66321791214601E-16,
1.)) ;
#36598=DIRECTION('ref_axis',(1.75658099177411E-13,1.,1.66321791206623E-16)) ;
#36599=DIRECTION('',(-1.75658099177411E-13,-1.,-1.66321791206623E-16)) ;
#36600=DIRECTION('center_axis',(4.54195640846217E-14,-1.66321791214601E-16,
1.)) ;
#36601=DIRECTION('ref_axis',(1.75658099177411E-13,1.,1.66321791206623E-16)) ;
#36602=DIRECTION('',(-1.75658099177411E-13,-1.,-1.66321791206623E-16)) ;
#36603=DIRECTION('center_axis',(4.54195640846217E-14,-1.66321791214601E-16,
1.)) ;
#36604=DIRECTION('ref_axis',(1.75658099177411E-13,1.,1.66321791206623E-16)) ;
#36605=DIRECTION('',(1.75658099177411E-13,1.,1.66321791206623E-16)) ;
#36606=DIRECTION('center_axis',(4.54195640846217E-14,-1.66321791214601E-16,
1.)) ;
#36607=DIRECTION('ref_axis',(1.75658099177411E-13,1.,1.66321791206623E-16)) ;
#36608=DIRECTION('center_axis',(4.54195640846217E-14,-1.66321791214601E-16,
1.)) ;
#36609=DIRECTION('ref_axis',(1.,-1.75824632631105E-13,-4.54195640846217E-14)) ;
#36610=DIRECTION('center_axis',(4.54195640846217E-14,-1.66321791214601E-16,
1.)) ;
#36611=DIRECTION('ref_axis',(1.,-1.75824632631105E-13,-4.54195640846217E-14)) ;
#36612=DIRECTION('center_axis',(4.54195640846217E-14,-1.66321791214601E-16,
1.)) ;
#36613=DIRECTION('ref_axis',(0.707106781186672,0.707106781186423,-3.19988744963517E-14)) ;
#36614=DIRECTION('center_axis',(4.54195640846217E-14,-1.66321791214601E-16,
1.)) ;
#36615=DIRECTION('ref_axis',(0.707106781186672,0.707106781186423,-3.19988744963517E-14)) ;
#36616=DIRECTION('center_axis',(4.54195640846217E-14,-1.66321791214601E-16,
1.)) ;
#36617=DIRECTION('ref_axis',(0.707106781186672,0.707106781186423,-3.19988744963517E-14)) ;
#36618=DIRECTION('center_axis',(4.54195640846217E-14,-1.66321791214601E-16,
1.)) ;
#36619=DIRECTION('ref_axis',(0.707106781186672,0.707106781186423,-3.19988744963517E-14)) ;
#36620=DIRECTION('center_axis',(4.54195640846217E-14,-1.66321791214601E-16,
1.)) ;
#36621=DIRECTION('ref_axis',(-0.258819045102691,-0.965925826289023,1.15947936917534E-14)) ;
#36622=DIRECTION('center_axis',(4.54195640846217E-14,-1.66321791214601E-16,
1.)) ;
#36623=DIRECTION('ref_axis',(-1.75780563857326E-13,-1.,-1.66321791206617E-16)) ;
#36624=DIRECTION('center_axis',(4.54195640846217E-14,-1.66321791214601E-16,
1.)) ;
#36625=DIRECTION('ref_axis',(0.258819045102351,-0.965925826289114,-1.19161027189557E-14)) ;
#36626=DIRECTION('center_axis',(4.54195640846217E-14,-1.66321791214601E-16,
1.)) ;
#36627=DIRECTION('ref_axis',(-1.75780563857326E-13,-1.,-1.66321791206617E-16)) ;
#36628=DIRECTION('center_axis',(4.54195640846217E-14,-1.66321791214601E-16,
1.)) ;
#36629=DIRECTION('ref_axis',(0.965925826289023,-0.258819045102691,-4.39149772153074E-14)) ;
#36630=DIRECTION('center_axis',(4.54195640846217E-14,-1.66321791214601E-16,
1.)) ;
#36631=DIRECTION('ref_axis',(1.,-1.75841796197283E-13,-4.54195640846217E-14)) ;
#36632=DIRECTION('center_axis',(4.54195640846217E-14,-1.66321791214601E-16,
1.)) ;
#36633=DIRECTION('ref_axis',(0.965925826289114,0.258819045102351,-4.38288827209477E-14)) ;
#36634=DIRECTION('center_axis',(4.54195640846217E-14,-1.66321791214601E-16,
1.)) ;
#36635=DIRECTION('ref_axis',(1.,-1.75841796197283E-13,-4.54195640846217E-14)) ;
#36636=DIRECTION('center_axis',(4.54195640846217E-14,-1.66321791214601E-16,
1.)) ;
#36637=DIRECTION('ref_axis',(0.258819045102691,0.965925826289023,-1.15947936917534E-14)) ;
#36638=DIRECTION('center_axis',(4.54195640846217E-14,-1.66321791214601E-16,
1.)) ;
#36639=DIRECTION('ref_axis',(1.7590302853724E-13,1.,1.66321791206612E-16)) ;
#36640=DIRECTION('center_axis',(4.54195640846217E-14,-1.66321791214601E-16,
1.)) ;
#36641=DIRECTION('ref_axis',(-0.258819045102351,0.965925826289114,1.19161027189557E-14)) ;
#36642=DIRECTION('center_axis',(4.54195640846217E-14,-1.66321791214601E-16,
1.)) ;
#36643=DIRECTION('ref_axis',(1.7590302853724E-13,1.,1.66321791206612E-16)) ;
#36644=DIRECTION('center_axis',(4.54195640846217E-14,-1.66321791214601E-16,
1.)) ;
#36645=DIRECTION('ref_axis',(0.499999999999848,-0.866025403784527,-2.28538209386987E-14)) ;
#36646=DIRECTION('center_axis',(-4.54195640846217E-14,1.66321791214601E-16,
-1.)) ;
#36647=DIRECTION('ref_axis',(0.156305321293456,-0.987708786300572,-7.26359705179142E-15)) ;
#36648=DIRECTION('center_axis',(4.54195640846217E-14,-1.66321791214601E-16,
1.)) ;
#36649=DIRECTION('ref_axis',(-1.,5.55236256206829E-46,4.54195640846217E-14)) ;
#36650=DIRECTION('center_axis',(-4.54195640846217E-14,1.66321791214601E-16,
-1.)) ;
#36651=DIRECTION('ref_axis',(-0.987708878702966,0.156304737392474,4.48873035970976E-14)) ;
#36652=DIRECTION('center_axis',(-1.75658099177411E-13,-1.,-1.66321791206623E-16)) ;
#36653=DIRECTION('ref_axis',(-0.707106781186542,1.24091425832264E-13,0.707106781186553)) ;
#36654=DIRECTION('center_axis',(1.75658099177411E-13,1.,1.66321791206623E-16)) ;
#36655=DIRECTION('ref_axis',(-0.707106781186542,1.24091425832264E-13,0.707106781186553)) ;
#36656=DIRECTION('center_axis',(-1.75658099177411E-13,-1.,-1.66321791206623E-16)) ;
#36657=DIRECTION('ref_axis',(-0.707106781186542,1.24091425832264E-13,0.707106781186553)) ;
#36658=DIRECTION('',(1.75658099177411E-13,1.,1.66321791206623E-16)) ;
#36659=DIRECTION('center_axis',(-1.,1.75658099177411E-13,4.54195640846217E-14)) ;
#36660=DIRECTION('ref_axis',(-9.20925513358884E-14,-0.707106781186434,0.707106781186661)) ;
#36661=DIRECTION('center_axis',(1.,-1.75658099177411E-13,-4.54195640846217E-14)) ;
#36662=DIRECTION('ref_axis',(-9.20925513358884E-14,-0.707106781186434,0.707106781186661)) ;
#36663=DIRECTION('',(-1.,1.75658099177411E-13,4.54195640846217E-14)) ;
#36664=DIRECTION('center_axis',(-1.,1.75658099177411E-13,4.54195640846217E-14)) ;
#36665=DIRECTION('ref_axis',(-9.20925513358884E-14,-0.707106781186434,0.707106781186661)) ;
#36666=DIRECTION('center_axis',(1.75658099177411E-13,1.,1.66321791206623E-16)) ;
#36667=DIRECTION('ref_axis',(-4.54195640846217E-14,1.66321791214601E-16,
-1.)) ;
#36668=DIRECTION('',(4.54195640846217E-14,-1.66321791214601E-16,1.)) ;
#36669=DIRECTION('center_axis',(-1.75658099177411E-13,-1.,-1.66321791206623E-16)) ;
#36670=DIRECTION('ref_axis',(0.70710678118651,-1.24091425832259E-13,-0.707106781186585)) ;
#36671=DIRECTION('',(1.,-1.75658099177411E-13,-4.53796366499639E-14)) ;
#36672=DIRECTION('center_axis',(1.75658099177411E-13,1.,1.66321791206623E-16)) ;
#36673=DIRECTION('ref_axis',(-0.707106781186529,1.24091425832262E-13,0.707106781186566)) ;
#36674=DIRECTION('',(-2.98822568073276E-29,-1.66321791206623E-16,1.)) ;
#36675=DIRECTION('center_axis',(-1.75658099177411E-13,-1.,-1.66321791206623E-16)) ;
#36676=DIRECTION('ref_axis',(0.707106781186551,-1.24091425832266E-13,-0.707106781186544)) ;
#36677=DIRECTION('',(1.,-1.75658099177411E-13,-4.54195640846217E-14)) ;
#36678=DIRECTION('center_axis',(-1.75658099177411E-13,-1.,-1.66321791206623E-16)) ;
#36679=DIRECTION('ref_axis',(-0.707106781186579,1.24326640365113E-13,-0.707106781186516)) ;
#36680=DIRECTION('',(2.92172610985041E-29,1.66321791206623E-16,-1.)) ;
#36681=DIRECTION('center_axis',(1.75658099177411E-13,1.,1.66321791206623E-16)) ;
#36682=DIRECTION('ref_axis',(0.707106781186554,-1.24326640365109E-13,0.707106781186541)) ;
#36683=DIRECTION('',(1.,-1.75658099177411E-13,-4.54224185797219E-14)) ;
#36684=DIRECTION('center_axis',(1.75658099177411E-13,1.,1.66321791206623E-16)) ;
#36685=DIRECTION('ref_axis',(-0.707106781186538,1.24091425832263E-13,0.707106781186557)) ;
#36686=DIRECTION('',(-2.92157696951376E-29,-1.66321791206623E-16,1.)) ;
#36687=DIRECTION('center_axis',(-1.75658099177411E-13,-1.,-1.66321791206623E-16)) ;
#36688=DIRECTION('ref_axis',(0.707106781186529,-1.24091425832262E-13,-0.707106781186566)) ;
#36689=DIRECTION('',(1.,-1.75658099177411E-13,-4.54195640846217E-14)) ;
#36690=DIRECTION('center_axis',(-1.75658099177411E-13,-1.,-1.66321791206623E-16)) ;
#36691=DIRECTION('ref_axis',(-0.70710678118658,1.24326640365113E-13,-0.707106781186515)) ;
#36692=DIRECTION('',(-4.54195640846217E-14,1.66321791214601E-16,-1.)) ;
#36693=DIRECTION('center_axis',(1.75658099177411E-13,1.,1.66321791206623E-16)) ;
#36694=DIRECTION('ref_axis',(-1.,1.75658099177411E-13,1.34042507393854E-33)) ;
#36695=DIRECTION('center_axis',(1.75658099177411E-13,1.,1.66321791206623E-16)) ;
#36696=DIRECTION('ref_axis',(-1.,1.75658099177411E-13,6.92942826962939E-35)) ;
#36697=DIRECTION('center_axis',(-1.,1.75658099177411E-13,4.54195640846217E-14)) ;
#36698=DIRECTION('ref_axis',(1.56325514861461E-13,0.70710678118656,0.707106781186535)) ;
#36699=DIRECTION('center_axis',(1.,-1.75658099177411E-13,-4.54195640846217E-14)) ;
#36700=DIRECTION('ref_axis',(1.56325514861461E-13,0.70710678118656,0.707106781186535)) ;
#36701=DIRECTION('',(1.,-1.75658099177411E-13,-4.54195640846217E-14)) ;
#36702=DIRECTION('center_axis',(-1.,1.75658099177411E-13,4.54195640846217E-14)) ;
#36703=DIRECTION('ref_axis',(1.56325514861461E-13,0.70710678118656,0.707106781186535)) ;
#36704=DIRECTION('',(-1.,1.75658099177411E-13,4.54195640846217E-14)) ;
#36705=DIRECTION('center_axis',(1.,-1.75658099177411E-13,-4.54195640846217E-14)) ;
#36706=DIRECTION('ref_axis',(1.75658099177411E-13,1.,1.66321791206623E-16)) ;
#36707=DIRECTION('',(4.54195640846217E-14,-1.66321791214601E-16,1.)) ;
#36708=DIRECTION('',(1.75658099177411E-13,1.,0.)) ;
#36709=DIRECTION('',(-4.54195640846217E-14,1.66321791214601E-16,-1.)) ;
#36710=DIRECTION('',(4.54195640846217E-14,-1.66321791214601E-16,1.)) ;
#36711=DIRECTION('',(-1.75658099177411E-13,-1.,-1.66321791206623E-16)) ;
#36712=DIRECTION('center_axis',(-1.75658099177411E-13,-1.,-1.66321791206623E-16)) ;
#36713=DIRECTION('ref_axis',(-2.33866651370291E-30,1.66321791206623E-16,
-1.)) ;
#36714=DIRECTION('',(-4.54195640846217E-14,1.66321791214601E-16,-1.)) ;
#36715=DIRECTION('center_axis',(-1.75658099177411E-13,-1.,-1.66321791206623E-16)) ;
#36716=DIRECTION('ref_axis',(0.70710678118651,-1.24091425832259E-13,-0.707106781186585)) ;
#36717=DIRECTION('',(1.,-1.75658099177411E-13,-4.54195640846217E-14)) ;
#36718=DIRECTION('center_axis',(1.75658099177411E-13,1.,1.66321791206623E-16)) ;
#36719=DIRECTION('ref_axis',(-0.707106781186529,1.24091425832262E-13,0.707106781186566)) ;
#36720=DIRECTION('',(1.32744277756511E-27,7.55696881488181E-15,1.)) ;
#36721=DIRECTION('center_axis',(-1.75658099177411E-13,-1.,-1.66321791206623E-16)) ;
#36722=DIRECTION('ref_axis',(0.707106781186551,-1.24091425832266E-13,-0.707106781186544)) ;
#36723=DIRECTION('',(-1.,1.75658099177411E-13,0.)) ;
#36724=DIRECTION('center_axis',(-1.75658099177411E-13,-1.,-1.66321791206623E-16)) ;
#36725=DIRECTION('ref_axis',(-0.707106781186551,1.24326640365108E-13,-0.707106781186544)) ;
#36726=DIRECTION('',(-1.32744277756505E-27,-7.55696881488144E-15,-1.)) ;
#36727=DIRECTION('center_axis',(1.75658099177411E-13,1.,1.66321791206623E-16)) ;
#36728=DIRECTION('ref_axis',(0.707106781186551,-1.24326640365108E-13,0.707106781186544)) ;
#36729=DIRECTION('',(1.,-1.75658099177411E-13,-4.54195640846217E-14)) ;
#36730=DIRECTION('center_axis',(1.75658099177411E-13,1.,1.66321791206623E-16)) ;
#36731=DIRECTION('ref_axis',(-0.707106781186535,1.24091425832263E-13,0.70710678118656)) ;
#36732=DIRECTION('',(2.92157696951376E-29,1.66321791206623E-16,-1.)) ;
#36733=DIRECTION('center_axis',(-1.75658099177411E-13,-1.,-1.66321791206623E-16)) ;
#36734=DIRECTION('ref_axis',(0.707106781186549,-1.24091425832265E-13,-0.707106781186546)) ;
#36735=DIRECTION('',(1.,-1.75658099177411E-13,-4.54195640846217E-14)) ;
#36736=DIRECTION('center_axis',(-1.75658099177411E-13,-1.,-1.66321791206623E-16)) ;
#36737=DIRECTION('ref_axis',(-0.707106781186561,1.2432664036511E-13,-0.707106781186534)) ;
#36738=DIRECTION('center_axis',(1.75658099177411E-13,1.,1.66321791206623E-16)) ;
#36739=DIRECTION('ref_axis',(0.99999997726804,-1.75658059720777E-13,-0.000213222701069828)) ;
#36740=DIRECTION('center_axis',(-1.75658099177411E-13,-1.,-1.66321791206623E-16)) ;
#36741=DIRECTION('ref_axis',(-1.,1.75658099177411E-13,-8.27097305203856E-32)) ;
#36742=DIRECTION('center_axis',(1.,-1.75658099177411E-13,-4.54195640846217E-14)) ;
#36743=DIRECTION('ref_axis',(-9.20925513359162E-14,-0.70710678118656,0.707106781186535)) ;
#36744=DIRECTION('center_axis',(-1.,1.75658099177411E-13,4.54195640846217E-14)) ;
#36745=DIRECTION('ref_axis',(-9.20925513359162E-14,-0.70710678118656,0.707106781186535)) ;
#36746=DIRECTION('',(-1.,1.75658099177411E-13,4.54195640846217E-14)) ;
#36747=DIRECTION('center_axis',(1.,-1.75658099177411E-13,-4.54195640846217E-14)) ;
#36748=DIRECTION('ref_axis',(-9.20925513359162E-14,-0.70710678118656,0.707106781186535)) ;
#36749=DIRECTION('',(1.,-1.75658099177411E-13,-4.54195640846217E-14)) ;
#36750=DIRECTION('center_axis',(-1.,1.75658099177411E-13,4.54195640846217E-14)) ;
#36751=DIRECTION('ref_axis',(-1.75658099177411E-13,-1.,-1.66321791206623E-16)) ;
#36752=DIRECTION('',(4.54195640846217E-14,-1.66321791214601E-16,1.)) ;
#36753=DIRECTION('',(-1.75658099177411E-13,-1.,-1.81854713288318E-16)) ;
#36754=DIRECTION('',(-4.54195640846217E-14,1.66321791214601E-16,-1.)) ;
#36755=DIRECTION('',(1.75658099177411E-13,1.,1.66321791206623E-16)) ;
#36756=DIRECTION('center_axis',(1.75658099177411E-13,1.,1.66321791206623E-16)) ;
#36757=DIRECTION('ref_axis',(-4.54195640846217E-14,1.66321791214601E-16,
-1.)) ;
#36758=DIRECTION('',(4.54195640846217E-14,-1.66321791214601E-16,1.)) ;
#36759=DIRECTION('center_axis',(1.75658099177411E-13,1.,1.66321791206623E-16)) ;
#36760=DIRECTION('ref_axis',(-0.70710678118658,1.24326640365113E-13,-0.707106781186515)) ;
#36761=DIRECTION('',(-1.,1.75658099177411E-13,4.54195640846217E-14)) ;
#36762=DIRECTION('center_axis',(1.75658099177411E-13,1.,1.66321791206623E-16)) ;
#36763=DIRECTION('ref_axis',(0.707106781186529,-1.24091425832262E-13,-0.707106781186566)) ;
#36764=DIRECTION('',(-2.92157696951376E-29,-1.66321791206623E-16,1.)) ;
#36765=DIRECTION('center_axis',(-1.75658099177411E-13,-1.,-1.66321791206623E-16)) ;
#36766=DIRECTION('ref_axis',(-0.707106781186538,1.24091425832263E-13,0.707106781186557)) ;
#36767=DIRECTION('',(1.,-1.75658099177411E-13,-4.54224185797219E-14)) ;
#36768=DIRECTION('center_axis',(-1.75658099177411E-13,-1.,-1.66321791206623E-16)) ;
#36769=DIRECTION('ref_axis',(0.707106781186554,-1.24326640365109E-13,0.707106781186541)) ;
#36770=DIRECTION('',(2.92172610985041E-29,1.66321791206623E-16,-1.)) ;
#36771=DIRECTION('center_axis',(1.75658099177411E-13,1.,1.66321791206623E-16)) ;
#36772=DIRECTION('ref_axis',(-0.707106781186579,1.24326640365113E-13,-0.707106781186516)) ;
#36773=DIRECTION('',(-1.,1.75658099177411E-13,4.54195640846217E-14)) ;
#36774=DIRECTION('center_axis',(1.75658099177411E-13,1.,1.66321791206623E-16)) ;
#36775=DIRECTION('ref_axis',(0.707106781186551,-1.24091425832266E-13,-0.707106781186544)) ;
#36776=DIRECTION('',(-2.98822568073276E-29,-1.66321791206623E-16,1.)) ;
#36777=DIRECTION('center_axis',(-1.75658099177411E-13,-1.,-1.66321791206623E-16)) ;
#36778=DIRECTION('ref_axis',(-0.707106781186529,1.24091425832262E-13,0.707106781186566)) ;
#36779=DIRECTION('',(1.,-1.75658099177411E-13,-4.53796366499639E-14)) ;
#36780=DIRECTION('center_axis',(1.75658099177411E-13,1.,1.66321791206623E-16)) ;
#36781=DIRECTION('ref_axis',(0.70710678118651,-1.24091425832259E-13,-0.707106781186585)) ;
#36782=DIRECTION('center_axis',(1.75658099177411E-13,1.,1.66321791206623E-16)) ;
#36783=DIRECTION('ref_axis',(-1.,1.75658099177411E-13,1.34042507393854E-33)) ;
#36784=DIRECTION('center_axis',(1.75658099177411E-13,1.,1.66321791206623E-16)) ;
#36785=DIRECTION('ref_axis',(-1.,1.75658099177411E-13,6.92942826962939E-35)) ;
#36786=DIRECTION('center_axis',(-1.75744394921826E-13,-1.,-1.81854713288314E-16)) ;
#36787=DIRECTION('ref_axis',(-0.707106781186529,1.2414146270379E-13,0.707106781186566)) ;
#36788=DIRECTION('',(-1.75744394921826E-13,-1.,-1.81854713288314E-16)) ;
#36789=DIRECTION('center_axis',(-1.75658099177411E-13,-1.,-1.66321791206623E-16)) ;
#36790=DIRECTION('ref_axis',(-0.707106781186529,1.24091425832262E-13,0.707106781186566)) ;
#36791=DIRECTION('',(1.75744394921826E-13,1.,1.81854713288314E-16)) ;
#36792=DIRECTION('center_axis',(4.53796366499638E-14,-1.81854713296289E-16,
1.)) ;
#36793=DIRECTION('ref_axis',(-1.,1.75658099177411E-13,4.53796366499638E-14)) ;
#36794=DIRECTION('',(1.75658099177411E-13,1.,1.66321791206623E-16)) ;
#36795=DIRECTION('',(1.,-1.75658099177411E-13,-4.54195640846217E-14)) ;
#36796=DIRECTION('center_axis',(-1.75744394921826E-13,-1.,-1.81854713288314E-16)) ;
#36797=DIRECTION('ref_axis',(-0.707106781186529,1.2414146270379E-13,0.707106781186566)) ;
#36798=DIRECTION('',(-1.75744394921826E-13,-1.,-1.81854713288314E-16)) ;
#36799=DIRECTION('',(1.75744394921826E-13,1.,1.81854713288314E-16)) ;
#36800=DIRECTION('center_axis',(4.53796366499638E-14,-1.81854713296289E-16,
1.)) ;
#36801=DIRECTION('ref_axis',(-1.,1.75658099177411E-13,4.53796366499638E-14)) ;
#36802=DIRECTION('',(1.75658099177411E-13,1.,1.81854713288318E-16)) ;
#36803=DIRECTION('center_axis',(-1.75658099177411E-13,-1.,-1.66321791206623E-16)) ;
#36804=DIRECTION('ref_axis',(-0.707106781186507,1.24091425832258E-13,0.707106781186588)) ;
#36805=DIRECTION('center_axis',(1.75658099177411E-13,1.,1.66321791206623E-16)) ;
#36806=DIRECTION('ref_axis',(-0.707106781186507,1.24091425832258E-13,0.707106781186588)) ;
#36807=DIRECTION('',(1.75658099177411E-13,1.,1.66321791206623E-16)) ;
#36808=DIRECTION('center_axis',(-1.75658099177411E-13,-1.,-1.66321791206623E-16)) ;
#36809=DIRECTION('ref_axis',(-0.707106781186507,1.24091425832258E-13,0.707106781186588)) ;
#36810=DIRECTION('',(-1.75658099177411E-13,-1.,-1.66321791206623E-16)) ;
#36811=DIRECTION('center_axis',(-1.75658099177411E-13,-1.,-1.66321791206623E-16)) ;
#36812=DIRECTION('ref_axis',(1.,-1.75658099177411E-13,-4.54195640846217E-14)) ;
#36813=DIRECTION('',(-1.,1.75658099177411E-13,4.54195640846217E-14)) ;
#36814=DIRECTION('',(-4.54195640846217E-14,1.66321791214601E-16,-1.)) ;
#36815=DIRECTION('',(1.,-1.75658099177411E-13,-4.54195640846217E-14)) ;
#36816=DIRECTION('',(4.54195640846217E-14,-1.66321791214601E-16,1.)) ;
#36817=DIRECTION('center_axis',(4.54195640846217E-14,-1.66321791214601E-16,
1.)) ;
#36818=DIRECTION('ref_axis',(1.,-1.75658099177411E-13,-4.54195640846217E-14)) ;
#36819=DIRECTION('',(1.,-1.75658099177411E-13,-4.54195640846217E-14)) ;
#36820=DIRECTION('',(1.35690070290911E-13,1.,1.66321791208438E-16)) ;
#36821=DIRECTION('',(-1.,5.13165898663611E-13,4.00690931964822E-13)) ;
#36822=DIRECTION('',(-1.75658099177411E-13,-1.,-1.66321791206623E-16)) ;
#36823=DIRECTION('',(1.,-1.75658099177411E-13,-4.36218068752822E-13)) ;
#36824=DIRECTION('',(-4.59875193481411E-13,-1.,-1.66321791193714E-16)) ;
#36825=DIRECTION('center_axis',(4.54195640846217E-14,-1.66321791214601E-16,
1.)) ;
#36826=DIRECTION('ref_axis',(0.707106781186423,-0.707106781186672,-3.22340890291943E-14)) ;
#36827=DIRECTION('center_axis',(4.54195640846217E-14,-1.66321791214601E-16,
1.)) ;
#36828=DIRECTION('ref_axis',(-0.987708878702966,0.156304737392474,4.48873035970976E-14)) ;
#36829=DIRECTION('center_axis',(4.54195640846217E-14,-1.66321791214601E-16,
1.)) ;
#36830=DIRECTION('ref_axis',(-1.,5.55236256206829E-46,4.54195640846217E-14)) ;
#36831=DIRECTION('center_axis',(4.54195640846217E-14,-1.66321791214601E-16,
1.)) ;
#36832=DIRECTION('ref_axis',(0.156305321293456,-0.987708786300572,-7.26359705179142E-15)) ;
#36833=DIRECTION('center_axis',(-4.54195640846217E-14,1.66321791214621E-16,
-1.)) ;
#36834=DIRECTION('ref_axis',(1.,1.87077983243537E-9,-4.54195640843106E-14)) ;
#36835=DIRECTION('center_axis',(-4.54195640846217E-14,1.66321791214621E-16,
-1.)) ;
#36836=DIRECTION('ref_axis',(1.,1.75488086631674E-8,-4.54195640817029E-14)) ;
#36837=DIRECTION('center_axis',(-4.54195640846217E-14,1.66321791214601E-16,
-1.)) ;
#36838=DIRECTION('ref_axis',(-1.,2.41975421181691E-13,4.54195640846217E-14)) ;
#36839=DIRECTION('',(1.75658099177411E-13,1.,1.66321791206623E-16)) ;
#36840=DIRECTION('center_axis',(-4.54195640846217E-14,1.66321791214601E-16,
-1.)) ;
#36841=DIRECTION('ref_axis',(1.,-9.98668740296709E-14,-4.54195640846217E-14)) ;
#36842=DIRECTION('',(-1.75658099177411E-13,-1.,-1.66321791206623E-16)) ;
#36843=DIRECTION('center_axis',(-4.54195640846217E-14,1.66321791214601E-16,
-1.)) ;
#36844=DIRECTION('ref_axis',(-1.,2.41975421181691E-13,4.54195640846217E-14)) ;
#36845=DIRECTION('',(1.75658099177411E-13,1.,1.66321791206623E-16)) ;
#36846=DIRECTION('center_axis',(-4.54195640846217E-14,1.66321791214601E-16,
-1.)) ;
#36847=DIRECTION('ref_axis',(1.,-9.98668740296709E-14,-4.54195640846217E-14)) ;
#36848=DIRECTION('',(-1.75658099177411E-13,-1.,-1.66321791206623E-16)) ;
#36849=DIRECTION('center_axis',(-4.54195640846217E-14,1.66321791214601E-16,
-1.)) ;
#36850=DIRECTION('ref_axis',(-1.,2.41975421181691E-13,4.54195640846217E-14)) ;
#36851=DIRECTION('',(1.75658099177411E-13,1.,1.66321791206623E-16)) ;
#36852=DIRECTION('center_axis',(-4.54195640846217E-14,1.66321791214601E-16,
-1.)) ;
#36853=DIRECTION('ref_axis',(1.,-9.98668740296709E-14,-4.54195640846217E-14)) ;
#36854=DIRECTION('',(-1.75658099177411E-13,-1.,-1.66321791206623E-16)) ;
#36855=DIRECTION('center_axis',(-4.54195640846217E-14,1.66321791214601E-16,
-1.)) ;
#36856=DIRECTION('ref_axis',(-1.,2.41975421181691E-13,4.54195640846217E-14)) ;
#36857=DIRECTION('',(1.75658099177411E-13,1.,1.66321791206623E-16)) ;
#36858=DIRECTION('center_axis',(-4.54195640846217E-14,1.66321791214601E-16,
-1.)) ;
#36859=DIRECTION('ref_axis',(1.,-1.09340777173131E-13,-4.54195640846217E-14)) ;
#36860=DIRECTION('',(-1.75658099177411E-13,-1.,-1.66321791206623E-16)) ;
#36861=DIRECTION('center_axis',(-4.54195640846217E-14,1.66321791214601E-16,
-1.)) ;
#36862=DIRECTION('ref_axis',(1.,-1.09340777173131E-13,-4.54195640846217E-14)) ;
#36863=DIRECTION('',(-1.75658099177411E-13,-1.,-1.66321791206623E-16)) ;
#36864=DIRECTION('center_axis',(-4.54195640846217E-14,1.66321791214601E-16,
-1.)) ;
#36865=DIRECTION('ref_axis',(-1.,2.41975421181691E-13,4.54195640846217E-14)) ;
#36866=DIRECTION('',(1.75658099177411E-13,1.,1.66321791206623E-16)) ;
#36867=DIRECTION('center_axis',(-4.54195640846217E-14,1.66321791214601E-16,
-1.)) ;
#36868=DIRECTION('ref_axis',(-1.,2.41975421181691E-13,4.54195640846217E-14)) ;
#36869=DIRECTION('',(1.75658099177411E-13,1.,1.66321791206623E-16)) ;
#36870=DIRECTION('center_axis',(-4.54195640846217E-14,1.66321791214601E-16,
-1.)) ;
#36871=DIRECTION('ref_axis',(1.,-1.09340777173131E-13,-4.54195640846217E-14)) ;
#36872=DIRECTION('',(-1.75658099177411E-13,-1.,-1.66321791206623E-16)) ;
#36873=DIRECTION('center_axis',(-4.54195640846217E-14,1.66321791214608E-16,
-1.)) ;
#36874=DIRECTION('ref_axis',(0.707106781186672,0.707106781186423,-3.19988744963517E-14)) ;
#36875=DIRECTION('center_axis',(-4.54195640846217E-14,1.66321791214608E-16,
-1.)) ;
#36876=DIRECTION('ref_axis',(0.707106781186679,0.707106781186416,-3.1998874496352E-14)) ;
#36877=DIRECTION('center_axis',(-4.54195640846217E-14,1.66321791214608E-16,
-1.)) ;
#36878=DIRECTION('ref_axis',(-0.707106781186672,-0.707106781186423,3.19988744963517E-14)) ;
#36879=DIRECTION('center_axis',(-4.54195640846217E-14,1.66321791214608E-16,
-1.)) ;
#36880=DIRECTION('ref_axis',(-0.707106781186649,-0.707106781186446,3.19988744963507E-14)) ;
#36881=DIRECTION('center_axis',(1.10810639983346E-16,4.54750752358529E-14,
1.)) ;
#36882=DIRECTION('ref_axis',(-1.,1.75719331517368E-13,1.10810639975355E-16)) ;
#36883=DIRECTION('center_axis',(4.54195640846217E-14,-1.66321791214601E-16,
1.)) ;
#36884=DIRECTION('ref_axis',(-0.965925826289114,-0.258819045102351,4.38288827209477E-14)) ;
#36885=DIRECTION('center_axis',(-4.54195640846217E-14,1.66321791214601E-16,
-1.)) ;
#36886=DIRECTION('ref_axis',(-1.,1.75719331517368E-13,4.54195640846217E-14)) ;
#36887=DIRECTION('center_axis',(4.54195640846217E-14,-1.66321791214601E-16,
1.)) ;
#36888=DIRECTION('ref_axis',(-0.965925826289023,0.25881904510269,4.39149772153074E-14)) ;
#36889=DIRECTION('center_axis',(4.54195640846217E-14,-1.66321791214602E-16,
1.)) ;
#36890=DIRECTION('ref_axis',(-0.258819045102691,-0.965925826289023,1.15947936917534E-14)) ;
#36891=DIRECTION('center_axis',(-2.21832942445859E-16,-4.54750752358529E-14,
1.)) ;
#36892=DIRECTION('ref_axis',(-1.75780563857328E-13,-1.,-4.54750752358529E-14)) ;
#36893=DIRECTION('center_axis',(4.54195640846217E-14,-1.66321791214602E-16,
1.)) ;
#36894=DIRECTION('ref_axis',(0.258819045102351,-0.965925826289114,-1.19161027189557E-14)) ;
#36895=DIRECTION('center_axis',(-4.54195640846217E-14,1.66321791214602E-16,
-1.)) ;
#36896=DIRECTION('ref_axis',(-1.75780563857326E-13,-1.,-1.66321791206618E-16)) ;
#36897=DIRECTION('center_axis',(4.54195640846217E-14,-1.66321791214601E-16,
1.)) ;
#36898=DIRECTION('ref_axis',(0.965925826289023,-0.258819045102691,-4.39149772153074E-14)) ;
#36899=DIRECTION('center_axis',(9.072831752926E-14,-4.58077188182821E-14,
1.)) ;
#36900=DIRECTION('ref_axis',(1.,-1.75841796197283E-13,-9.07283175292681E-14)) ;
#36901=DIRECTION('center_axis',(4.54195640846217E-14,-1.66321791214601E-16,
1.)) ;
#36902=DIRECTION('ref_axis',(0.965925826289114,0.258819045102351,-4.38288827209477E-14)) ;
#36903=DIRECTION('center_axis',(-4.54195640846217E-14,1.66321791214601E-16,
-1.)) ;
#36904=DIRECTION('ref_axis',(1.,-1.75841796197283E-13,-4.54195640846217E-14)) ;
#36905=DIRECTION('center_axis',(4.54195640846217E-14,-1.66321791214602E-16,
1.)) ;
#36906=DIRECTION('ref_axis',(0.258819045102691,0.965925826289023,-1.15947936917534E-14)) ;
#36907=DIRECTION('center_axis',(9.10609611116892E-14,4.51424316534237E-14,
1.)) ;
#36908=DIRECTION('ref_axis',(1.75903028537238E-13,1.,-4.51424316534397E-14)) ;
#36909=DIRECTION('center_axis',(4.54195640846217E-14,-1.66321791214602E-16,
1.)) ;
#36910=DIRECTION('ref_axis',(-0.258819045102351,0.965925826289114,1.19161027189557E-14)) ;
#36911=DIRECTION('center_axis',(-4.54195640846217E-14,1.66321791214602E-16,
-1.)) ;
#36912=DIRECTION('ref_axis',(1.7590302853724E-13,1.,1.66321791206613E-16)) ;
#36913=DIRECTION('center_axis',(4.54195640846217E-14,-1.66321791214602E-16,
1.)) ;
#36914=DIRECTION('ref_axis',(0.707106781186672,0.707106781186423,-3.19988744963517E-14)) ;
#36915=DIRECTION('center_axis',(4.54195640846217E-14,-1.66321791214601E-16,
1.)) ;
#36916=DIRECTION('ref_axis',(-0.156304737392422,-0.987708878702974,6.93501552682063E-15)) ;
#36917=DIRECTION('center_axis',(4.54195640846217E-14,-1.66321791214601E-16,
1.)) ;
#36918=DIRECTION('ref_axis',(-1.,5.55236256206829E-46,4.54195640846217E-14)) ;
#36919=DIRECTION('center_axis',(4.54195640846217E-14,-1.66321791214601E-16,
1.)) ;
#36920=DIRECTION('ref_axis',(0.987707474797848,0.156313608583704,-4.48352445890699E-14)) ;
#36921=DIRECTION('center_axis',(4.54195640846217E-14,-1.66321791214601E-16,
1.)) ;
#36922=DIRECTION('ref_axis',(-0.707106781186423,0.707106781186672,3.22340890291943E-14)) ;
#36923=DIRECTION('center_axis',(4.54195640846217E-14,-1.66321791214601E-16,
1.)) ;
#36924=DIRECTION('ref_axis',(0.987708878702962,-0.1563047373925,-4.48873035970975E-14)) ;
#36925=DIRECTION('center_axis',(4.54195640846217E-14,-1.66321791214601E-16,
1.)) ;
#36926=DIRECTION('ref_axis',(-1.,5.55236256206829E-46,4.54195640846217E-14)) ;
#36927=DIRECTION('center_axis',(4.54195640846217E-14,-1.66321791214602E-16,
1.)) ;
#36928=DIRECTION('ref_axis',(-0.707106781186672,-0.707106781186423,3.19988744963517E-14)) ;
#36929=DIRECTION('center_axis',(4.54195640846217E-14,-1.66321791214601E-16,
1.)) ;
#36930=DIRECTION('ref_axis',(0.156304737392435,0.987708878702972,-6.93501552682122E-15)) ;
#36931=DIRECTION('center_axis',(4.54195640846217E-14,-1.66321791214601E-16,
1.)) ;
#36932=DIRECTION('ref_axis',(-1.,5.55236256206829E-46,4.54195640846217E-14)) ;
#36933=DIRECTION('center_axis',(1.75658099177411E-13,1.,1.66321791206623E-16)) ;
#36934=DIRECTION('ref_axis',(-4.54195640846217E-14,1.66321791214601E-16,
-1.)) ;
#36935=DIRECTION('center_axis',(1.75658099177411E-13,1.,1.66321791206623E-16)) ;
#36936=DIRECTION('ref_axis',(-0.707106781186561,1.2432664036511E-13,-0.707106781186534)) ;
#36937=DIRECTION('',(-1.,1.75658099177411E-13,0.)) ;
#36938=DIRECTION('center_axis',(1.75658099177411E-13,1.,1.66321791206623E-16)) ;
#36939=DIRECTION('ref_axis',(0.707106781186549,-1.24091425832265E-13,-0.707106781186546)) ;
#36940=DIRECTION('',(2.92157696951376E-29,1.66321791206623E-16,-1.)) ;
#36941=DIRECTION('center_axis',(-1.75658099177411E-13,-1.,-1.66321791206623E-16)) ;
#36942=DIRECTION('ref_axis',(-0.707106781186535,1.24091425832263E-13,0.70710678118656)) ;
#36943=DIRECTION('',(1.,-1.75658099177411E-13,-4.54195640846217E-14)) ;
#36944=DIRECTION('center_axis',(-1.75658099177411E-13,-1.,-1.66321791206623E-16)) ;
#36945=DIRECTION('ref_axis',(0.707106781186551,-1.24326640365108E-13,0.707106781186544)) ;
#36946=DIRECTION('',(-1.35951365453452E-28,-1.66321791206623E-16,1.)) ;
#36947=DIRECTION('center_axis',(1.75658099177411E-13,1.,1.66321791206623E-16)) ;
#36948=DIRECTION('ref_axis',(-0.707106781186551,1.24326640365108E-13,-0.707106781186544)) ;
#36949=DIRECTION('',(-1.,1.75658099177411E-13,0.)) ;
#36950=DIRECTION('center_axis',(1.75658099177411E-13,1.,1.66321791206623E-16)) ;
#36951=DIRECTION('ref_axis',(0.707106781186551,-1.24091425832266E-13,-0.707106781186544)) ;
#36952=DIRECTION('',(1.35951365453457E-28,1.66321791206623E-16,-1.)) ;
#36953=DIRECTION('center_axis',(1.75658099177411E-13,1.,1.66321791206623E-16)) ;
#36954=DIRECTION('ref_axis',(0.70710678118651,-1.24091425832259E-13,-0.707106781186585)) ;
#36955=DIRECTION('',(4.54195640846217E-14,-1.66321791214601E-16,1.)) ;
#36956=DIRECTION('center_axis',(1.75658099177411E-13,1.,1.66321791206623E-16)) ;
#36957=DIRECTION('ref_axis',(0.99999997726804,-1.75658059720777E-13,-0.000213222701069828)) ;
#36958=DIRECTION('center_axis',(1.75658099177411E-13,1.,1.66321791206623E-16)) ;
#36959=DIRECTION('ref_axis',(-1.,1.75658099177411E-13,-8.27097305203856E-32)) ;
#36960=DIRECTION('center_axis',(1.,-1.75658099177411E-13,-4.54195640846217E-14)) ;
#36961=DIRECTION('ref_axis',(-4.54195640846217E-14,1.66321791214601E-16,
-1.)) ;
#36962=DIRECTION('',(4.54195640846217E-14,-1.66321791214601E-16,1.)) ;
#36963=DIRECTION('center_axis',(-1.,1.75658099177411E-13,4.54195640846217E-14)) ;
#36964=DIRECTION('ref_axis',(-1.56325514861457E-13,-0.707106781186529,-0.707106781186566)) ;
#36965=DIRECTION('',(-1.75658099177411E-13,-1.,-1.66321791206623E-16)) ;
#36966=DIRECTION('center_axis',(-1.,1.75658099177411E-13,4.54195640846217E-14)) ;
#36967=DIRECTION('ref_axis',(9.20925513359107E-14,0.707106781186535,-0.70710678118656)) ;
#36968=DIRECTION('center_axis',(6.65065844402311E-14,-2.78565702539647E-14,
1.)) ;
#36969=DIRECTION('ref_axis',(-0.987708878702966,0.156304737392474,7.00432578420257E-14)) ;
#36970=DIRECTION('',(4.44089209850064E-14,0.,1.)) ;
#36971=DIRECTION('',(5.41996232473793E-14,-2.07511428963625E-14,1.)) ;
#36972=DIRECTION('center_axis',(-4.44089209850064E-14,0.,-1.)) ;
#36973=DIRECTION('ref_axis',(-1.,0.,4.44089209850064E-14)) ;
#36974=DIRECTION('',(-4.44089209850064E-14,0.,-1.)) ;
#36975=DIRECTION('center_axis',(-5.83947887444131E-11,-9.23392314221282E-12,
-1.)) ;
#36976=DIRECTION('ref_axis',(0.987707474797848,0.156313608583704,-5.91203571798419E-11)) ;
#36977=DIRECTION('',(-4.44089209850062E-14,0.,-1.)) ;
#36978=DIRECTION('',(7.99435328682709E-14,4.25044929548771E-15,1.)) ;
#36979=DIRECTION('center_axis',(-4.44089209850062E-14,0.,-1.)) ;
#36980=DIRECTION('ref_axis',(-1.,0.,4.44089209850062E-14)) ;
#36981=DIRECTION('',(4.44089209850062E-14,0.,1.)) ;
#36982=DIRECTION('center_axis',(7.31098125473717E-14,2.09206985643948E-14,
1.)) ;
#36983=DIRECTION('ref_axis',(-0.156304737392422,-0.987708878702974,3.20909697717474E-14)) ;
#36984=DIRECTION('',(6.60043851897696E-14,8.613737371543E-15,1.)) ;
#36985=DIRECTION('',(-6.91631936757579E-11,4.36746934819318E-10,-1.)) ;
#36986=DIRECTION('',(6.94007814181027E-10,-4.38310128933186E-9,1.)) ;
#36987=DIRECTION('center_axis',(-4.44089209850062E-14,0.,-1.)) ;
#36988=DIRECTION('ref_axis',(-1.,0.,4.44089209850062E-14)) ;
#36989=DIRECTION('',(4.44089209850062E-14,0.,1.)) ;
#36990=DIRECTION('center_axis',(2.43325437290122E-14,2.75239266715355E-14,
1.)) ;
#36991=DIRECTION('ref_axis',(0.987708878702962,-0.1563047373925,-1.97313493521686E-14)) ;
#36992=DIRECTION('',(3.66395049218641E-14,2.04184993139333E-14,1.)) ;
#36993=DIRECTION('',(6.34499860060004E-10,1.00068101952864E-10,-1.)) ;
#36994=DIRECTION('',(5.64924462358365E-13,1.34783525161202E-13,1.)) ;
#36995=DIRECTION('center_axis',(-4.44089209850062E-14,0.,-1.)) ;
#36996=DIRECTION('ref_axis',(-1.,0.,4.44089209850062E-14)) ;
#36997=DIRECTION('',(4.44089209850062E-14,0.,1.)) ;
#36998=DIRECTION('center_axis',(1.77293156218716E-14,-2.1253342146824E-14,
1.)) ;
#36999=DIRECTION('ref_axis',(0.156304737392435,0.987708878702972,1.82209387181059E-14)) ;
#37000=DIRECTION('',(2.48347429794738E-14,-8.94638095397221E-15,1.)) ;
#37001=DIRECTION('center_axis',(-8.03175469292822E-12,5.04730250306102E-11,
-1.)) ;
#37002=DIRECTION('ref_axis',(0.156305321293456,-0.987708786300572,-5.11080562917308E-11)) ;
#37003=DIRECTION('',(-8.95302828677947E-14,5.19338576482528E-13,1.)) ;
#37004=DIRECTION('center_axis',(1.,-1.75658099177411E-13,-4.54195640846217E-14)) ;
#37005=DIRECTION('ref_axis',(9.20925513359107E-14,0.707106781186535,-0.70710678118656)) ;
#37006=DIRECTION('',(-1.,1.75658099177411E-13,4.54195640846217E-14)) ;
#37007=DIRECTION('center_axis',(1.,-1.75658099177411E-13,-4.54195640846217E-14)) ;
#37008=DIRECTION('ref_axis',(9.20925513359107E-14,0.707106781186535,-0.70710678118656)) ;
#37009=DIRECTION('center_axis',(4.54195640846217E-14,-1.66321791214601E-16,
1.)) ;
#37010=DIRECTION('ref_axis',(-1.,1.75658099177411E-13,4.54195640846217E-14)) ;
#37011=DIRECTION('',(1.,-1.75658099177411E-13,-4.54195640846217E-14)) ;
#37012=DIRECTION('',(1.75658099177411E-13,1.,1.66321791206623E-16)) ;
#37013=DIRECTION('center_axis',(1.,-1.75658099177411E-13,-4.54195640846217E-14)) ;
#37014=DIRECTION('ref_axis',(-1.56325514861457E-13,-0.707106781186529,-0.707106781186566)) ;
#37015=DIRECTION('',(-1.,1.75658099177411E-13,4.54195640846217E-14)) ;
#37016=DIRECTION('center_axis',(1.,-1.75658099177411E-13,-4.54195640846217E-14)) ;
#37017=DIRECTION('ref_axis',(-1.56325514861457E-13,-0.707106781186529,-0.707106781186566)) ;
#37018=DIRECTION('center_axis',(1.75658099177411E-13,1.,1.66321791206623E-16)) ;
#37019=DIRECTION('ref_axis',(-1.,1.75658099177411E-13,4.54195640846217E-14)) ;
#37020=DIRECTION('',(-4.54195640846217E-14,1.66321791214601E-16,-1.)) ;
#37021=DIRECTION('',(-4.54195640846217E-14,1.66321791214601E-16,-1.)) ;
#37022=DIRECTION('center_axis',(1.75658099177411E-13,1.,1.81854713288318E-16)) ;
#37023=DIRECTION('ref_axis',(0.70710678118651,-1.24080442397723E-13,-0.707106781186585)) ;
#37024=DIRECTION('center_axis',(-1.,1.75658099177411E-13,4.54195640846217E-14)) ;
#37025=DIRECTION('ref_axis',(-1.56325514861457E-13,-0.707106781186529,-0.707106781186566)) ;
#37026=DIRECTION('center_axis',(1.,-1.75658099177411E-13,-4.54195640846217E-14)) ;
#37027=DIRECTION('ref_axis',(-1.56325514861457E-13,-0.707106781186529,-0.707106781186566)) ;
#37028=DIRECTION('',(1.,-1.75658099177411E-13,-4.54195640846217E-14)) ;
#37029=DIRECTION('center_axis',(-1.,1.75658099177411E-13,4.54195640846217E-14)) ;
#37030=DIRECTION('ref_axis',(-1.56325514861457E-13,-0.707106781186529,-0.707106781186566)) ;
#37031=DIRECTION('',(-1.,1.75658099177411E-13,4.54195640846217E-14)) ;
#37032=DIRECTION('center_axis',(4.54195640846217E-14,-1.66321791214601E-16,
1.)) ;
#37033=DIRECTION('ref_axis',(-1.75658099177411E-13,-1.,-1.66321791206623E-16)) ;
#37034=DIRECTION('',(-1.75658099177411E-13,-1.,-1.66321791206623E-16)) ;
#37035=DIRECTION('',(-1.,1.75658099177411E-13,4.54195640846217E-14)) ;
#37036=DIRECTION('',(-1.75658099177411E-13,-1.,-1.66321791206623E-16)) ;
#37037=DIRECTION('center_axis',(1.,-1.75658099177411E-13,-4.54195640846217E-14)) ;
#37038=DIRECTION('ref_axis',(-4.54195640846217E-14,1.66321791214601E-16,
-1.)) ;
#37039=DIRECTION('',(4.54195640846217E-14,-1.66321791214601E-16,1.)) ;
#37040=DIRECTION('',(-1.75658099177411E-13,-1.,-1.66321791206623E-16)) ;
#37041=DIRECTION('',(-4.54195640846217E-14,1.66321791214601E-16,-1.)) ;
#37042=DIRECTION('center_axis',(1.,-1.75658099177411E-13,-4.54195640846217E-14)) ;
#37043=DIRECTION('ref_axis',(9.20925513359094E-14,0.707106781186529,-0.707106781186566)) ;
#37044=DIRECTION('center_axis',(1.,-1.75658099177411E-13,-4.54195640846217E-14)) ;
#37045=DIRECTION('ref_axis',(9.20925513359094E-14,0.707106781186529,-0.707106781186566)) ;
#37046=DIRECTION('center_axis',(-1.,1.75658099177411E-13,4.54195640846217E-14)) ;
#37047=DIRECTION('ref_axis',(9.20925513359094E-14,0.707106781186529,-0.707106781186566)) ;
#37048=DIRECTION('',(1.,-1.75658099177411E-13,-4.54195640846217E-14)) ;
#37049=DIRECTION('center_axis',(-1.75658099177411E-13,-1.,-1.66321791206623E-16)) ;
#37050=DIRECTION('ref_axis',(1.,-1.75658099177411E-13,-4.54195640846217E-14)) ;
#37051=DIRECTION('center_axis',(1.75658099177411E-13,1.,1.66321791206623E-16)) ;
#37052=DIRECTION('ref_axis',(8.33151766584917E-14,-1.66321791221258E-16,
1.)) ;
#37053=DIRECTION('',(-4.54195640846217E-14,1.66321791214601E-16,-1.)) ;
#37054=DIRECTION('center_axis',(1.75658099177411E-13,1.,1.66321791206623E-16)) ;
#37055=DIRECTION('ref_axis',(0.707106781186548,-1.24326640365108E-13,0.707106781186548)) ;
#37056=DIRECTION('',(4.54195640846217E-14,-1.66321791214601E-16,1.)) ;
#37057=DIRECTION('center_axis',(-1.75658099177411E-13,-1.,-1.66321791206623E-16)) ;
#37058=DIRECTION('ref_axis',(0.70710678118651,-1.24091425832259E-13,-0.707106781186585)) ;
#37059=DIRECTION('',(-1.75658099177411E-13,-1.,-1.66321791206623E-16)) ;
#37060=DIRECTION('center_axis',(-1.,1.75658099177411E-13,4.54195640846217E-14)) ;
#37061=DIRECTION('ref_axis',(-1.75658099177411E-13,-1.,-1.66321791206623E-16)) ;
#37062=DIRECTION('center_axis',(-1.75744394921826E-13,-1.,-1.66321791206619E-16)) ;
#37063=DIRECTION('ref_axis',(0.707106781186551,-1.24152446138329E-13,-0.707106781186544)) ;
#37064=DIRECTION('',(1.75744394921826E-13,1.,1.66321791206619E-16)) ;
#37065=DIRECTION('',(-1.75744394921826E-13,-1.,-1.66321791206619E-16)) ;
#37066=DIRECTION('center_axis',(4.54195640846217E-14,-1.66321791214601E-16,
1.)) ;
#37067=DIRECTION('ref_axis',(-1.,1.75658099177411E-13,4.54195640846217E-14)) ;
#37068=DIRECTION('',(-1.72252784426699E-13,-1.,-1.66321791206777E-16)) ;
#37069=DIRECTION('center_axis',(-1.72252784426699E-13,-1.,0.)) ;
#37070=DIRECTION('ref_axis',(0.707106781186554,-1.21801111946385E-13,0.707106781186541)) ;
#37071=DIRECTION('',(-1.72252784426699E-13,-1.,0.)) ;
#37072=DIRECTION('',(1.72252784426699E-13,1.,0.)) ;
#37073=DIRECTION('center_axis',(1.,-1.72252784426699E-13,5.67869452327227E-31)) ;
#37074=DIRECTION('ref_axis',(-2.92172610985041E-29,-1.66321791206623E-16,
1.)) ;
#37075=DIRECTION('',(1.72252784426699E-13,1.,1.66321791206777E-16)) ;
#37076=DIRECTION('center_axis',(1.72252784426699E-13,1.,1.66321791206777E-16)) ;
#37077=DIRECTION('ref_axis',(-0.707106781186579,1.2191871921281E-13,-0.707106781186516)) ;
#37078=DIRECTION('center_axis',(-1.72252784426699E-13,-1.,-1.66321791206777E-16)) ;
#37079=DIRECTION('ref_axis',(0.707106781186529,-1.21683504679959E-13,-0.707106781186566)) ;
#37080=DIRECTION('',(1.72252784426699E-13,1.,1.66321791206777E-16)) ;
#37081=DIRECTION('',(-1.72252784426699E-13,-1.,-1.66321791206777E-16)) ;
#37082=DIRECTION('center_axis',(4.54195640846217E-14,-1.66321791214601E-16,
1.)) ;
#37083=DIRECTION('ref_axis',(-1.,1.75658099177411E-13,4.54195640846217E-14)) ;
#37084=DIRECTION('',(-1.75658099177411E-13,-1.,-1.66321791206623E-16)) ;
#37085=DIRECTION('center_axis',(-1.72252784426699E-13,-1.,0.)) ;
#37086=DIRECTION('ref_axis',(-0.707106781186538,1.21801111946382E-13,0.707106781186557)) ;
#37087=DIRECTION('',(-1.72252784426699E-13,-1.,0.)) ;
#37088=DIRECTION('',(1.72252784426699E-13,1.,0.)) ;
#37089=DIRECTION('center_axis',(4.54224185797219E-14,-7.82413807575213E-27,
1.)) ;
#37090=DIRECTION('ref_axis',(-1.,1.75658099177411E-13,4.54224185797219E-14)) ;
#37091=DIRECTION('center_axis',(1.75658099177411E-13,1.,1.66321791206623E-16)) ;
#37092=DIRECTION('ref_axis',(-0.70710678118658,1.24326640365113E-13,-0.707106781186515)) ;
#37093=DIRECTION('',(1.75658099177411E-13,1.,1.66321791206623E-16)) ;
#37094=DIRECTION('center_axis',(1.7578531223231E-13,1.,1.66321791206617E-16)) ;
#37095=DIRECTION('ref_axis',(-0.707106781186535,1.24181379046037E-13,0.70710678118656)) ;
#37096=DIRECTION('',(1.7578531223231E-13,1.,1.66321791206617E-16)) ;
#37097=DIRECTION('',(-1.7578531223231E-13,-1.,-1.66321791206617E-16)) ;
#37098=DIRECTION('center_axis',(1.,-1.7578531223231E-13,-2.11583031556481E-32)) ;
#37099=DIRECTION('ref_axis',(-2.92157696951377E-29,-1.66321791206623E-16,
1.)) ;
#37100=DIRECTION('',(-1.7578531223231E-13,-1.,0.)) ;
#37101=DIRECTION('center_axis',(-1.7578531223231E-13,-1.,0.)) ;
#37102=DIRECTION('ref_axis',(0.707106781186549,-1.24298986312461E-13,-0.707106781186546)) ;
#37103=DIRECTION('',(1.7578531223231E-13,1.,0.)) ;
#37104=DIRECTION('center_axis',(0.,0.,-1.)) ;
#37105=DIRECTION('ref_axis',(1.,-1.75658099177411E-13,0.)) ;
#37106=DIRECTION('',(-1.75658099177411E-13,-1.,0.)) ;
#37107=DIRECTION('center_axis',(1.75658099177411E-13,1.,0.)) ;
#37108=DIRECTION('ref_axis',(-0.707106781186561,1.24209033098689E-13,-0.707106781186534)) ;
#37109=DIRECTION('center_axis',(-1.89478062869335E-13,-1.,-1.66321791205995E-16)) ;
#37110=DIRECTION('ref_axis',(0.707106781186551,-1.34098830407419E-13,0.707106781186544)) ;
#37111=DIRECTION('',(-1.89478062869335E-13,-1.,-1.66321791205995E-16)) ;
#37112=DIRECTION('',(1.89478062869335E-13,1.,1.66321791205995E-16)) ;
#37113=DIRECTION('center_axis',(-1.,1.89478062869335E-13,-1.04437034642664E-28)) ;
#37114=DIRECTION('ref_axis',(-1.32744277756505E-27,-7.55696881488144E-15,
-1.)) ;
#37115=DIRECTION('',(1.89478062869335E-13,1.,0.)) ;
#37116=DIRECTION('center_axis',(-1.89478062869335E-13,-1.,0.)) ;
#37117=DIRECTION('ref_axis',(-0.707106781186551,1.33981223140998E-13,-0.707106781186544)) ;
#37118=DIRECTION('',(-1.89478062869335E-13,-1.,0.)) ;
#37119=DIRECTION('center_axis',(-1.,1.75744394921826E-13,-6.52134249405362E-31)) ;
#37120=DIRECTION('ref_axis',(-1.32744277756511E-27,-7.55696881488181E-15,
-1.)) ;
#37121=DIRECTION('',(-1.89478062869335E-13,-1.,0.)) ;
#37122=DIRECTION('center_axis',(-1.89478062869335E-13,-1.,0.)) ;
#37123=DIRECTION('ref_axis',(0.707106781186551,-1.33981223140998E-13,-0.707106781186544)) ;
#37124=DIRECTION('',(1.89478062869335E-13,1.,0.)) ;
#37125=DIRECTION('center_axis',(0.,0.,-1.)) ;
#37126=DIRECTION('ref_axis',(1.,-1.75658099177411E-13,0.)) ;
#37127=DIRECTION('center_axis',(-1.75658099177411E-13,-1.,-1.66321791206623E-16)) ;
#37128=DIRECTION('ref_axis',(0.707106781186548,-1.24326640365108E-13,0.707106781186548)) ;
#37129=DIRECTION('center_axis',(-1.75658099177411E-13,-1.,-1.66321791206623E-16)) ;
#37130=DIRECTION('ref_axis',(0.707106781186548,-1.24326640365108E-13,0.707106781186548)) ;
#37131=DIRECTION('center_axis',(1.75658099177411E-13,1.,1.66321791206623E-16)) ;
#37132=DIRECTION('ref_axis',(-1.,1.75658099177411E-13,4.54195640846217E-14)) ;
#37133=DIRECTION('',(-4.54195640846217E-14,1.66321791214601E-16,-1.)) ;
#37134=DIRECTION('center_axis',(-1.75658099177411E-13,-1.,-1.66321791206623E-16)) ;
#37135=DIRECTION('ref_axis',(1.,-1.75658099177411E-13,9.19520314956783E-14)) ;
#37136=DIRECTION('center_axis',(1.,-1.75658099177411E-13,-4.54195640846217E-14)) ;
#37137=DIRECTION('ref_axis',(1.75658099177411E-13,1.,1.66321791206623E-16)) ;
#37138=DIRECTION('center_axis',(-1.,1.75744394921826E-13,-6.52134249405362E-31)) ;
#37139=DIRECTION('ref_axis',(-1.32744277756511E-27,-7.55696881488181E-15,
-1.)) ;
#37140=DIRECTION('center_axis',(-1.75662560300847E-13,-1.,-1.81854713288314E-16)) ;
#37141=DIRECTION('ref_axis',(-1.,1.75662560300847E-13,8.11276323366632E-34)) ;
#37142=DIRECTION('',(-1.75662560300847E-13,-1.,-1.81854713288314E-16)) ;
#37143=DIRECTION('center_axis',(-1.75744394921827E-13,-1.,-1.81854713288314E-16)) ;
#37144=DIRECTION('ref_axis',(-1.,1.75744394921827E-13,1.5693287858714E-32)) ;
#37145=DIRECTION('',(-1.75744394921827E-13,-1.,-1.81854713288314E-16)) ;
#37146=DIRECTION('center_axis',(-1.,1.72252784426699E-13,-5.66378048960696E-31)) ;
#37147=DIRECTION('ref_axis',(2.92157696951376E-29,1.66321791206623E-16,
-1.)) ;
#37148=DIRECTION('center_axis',(-1.76155386573851E-13,-1.,0.)) ;
#37149=DIRECTION('ref_axis',(-1.,1.76155386573851E-13,-4.62820191398731E-45)) ;
#37150=DIRECTION('',(-1.76155386573851E-13,-1.,0.)) ;
#37151=DIRECTION('center_axis',(1.34675317711724E-14,5.56466506464699E-14,
1.)) ;
#37152=DIRECTION('ref_axis',(0.529493733640589,0.848313848782011,-5.43367980621762E-14)) ;
#37153=DIRECTION('',(-7.72202224608625E-14,-2.9357493141945E-13,-1.)) ;
#37154=DIRECTION('',(2.44508561928056E-14,1.26579979998417E-14,-1.)) ;
#37155=DIRECTION('center_axis',(-1.01581938202089E-14,3.21931140438162E-14,
1.)) ;
#37156=DIRECTION('ref_axis',(0.52949373364028,-0.848313848782204,3.26885644516982E-14)) ;
#37157=DIRECTION('',(7.61868634881669E-14,-1.32198060448311E-13,-1.)) ;
#37158=DIRECTION('',(1.05568025685331E-13,-2.8988996425453E-13,1.)) ;
#37159=DIRECTION('center_axis',(1.10810639983346E-16,4.54750752358529E-14,
1.)) ;
#37160=DIRECTION('ref_axis',(-1.,1.75719331517368E-13,1.10810639975355E-16)) ;
#37161=DIRECTION('center_axis',(1.10810639983346E-16,4.54750752358529E-14,
1.)) ;
#37162=DIRECTION('ref_axis',(-1.,1.75719331517368E-13,1.10810639975355E-16)) ;
#37163=DIRECTION('center_axis',(4.10027929979194E-14,3.43576469924347E-14,
1.)) ;
#37164=DIRECTION('ref_axis',(-0.499999999999848,0.866025403784526,-9.253198610756E-15)) ;
#37165=DIRECTION('center_axis',(4.54195640846217E-14,-1.66321791214621E-16,
1.)) ;
#37166=DIRECTION('ref_axis',(1.,-1.75824632631105E-13,-4.54195640846217E-14)) ;
#37167=DIRECTION('',(-0.707106781186515,1.24122587161037E-13,0.70710678118658)) ;
#37168=DIRECTION('center_axis',(4.54195640846217E-14,-1.66321791214621E-16,
1.)) ;
#37169=DIRECTION('ref_axis',(1.,-1.75824632631105E-13,-4.54195640846217E-14)) ;
#37170=DIRECTION('',(-0.707106781186515,1.24122587161037E-13,0.70710678118658)) ;
#37171=DIRECTION('center_axis',(4.54195640846217E-14,-1.66321791214601E-16,
1.)) ;
#37172=DIRECTION('ref_axis',(-1.,1.75658099177411E-13,4.54195640846217E-14)) ;
#37173=DIRECTION('center_axis',(1.,-1.75658099177411E-13,-4.54195640846217E-14)) ;
#37174=DIRECTION('ref_axis',(-4.54195640846217E-14,0.,-1.)) ;
#37175=DIRECTION('center_axis',(4.54195640846217E-14,-1.66321791214608E-16,
1.)) ;
#37176=DIRECTION('ref_axis',(0.707106781186672,0.707106781186423,-3.19988744963517E-14)) ;
#37177=DIRECTION('',(4.54195640846217E-14,-1.66321791214608E-16,1.)) ;
#37178=DIRECTION('center_axis',(4.54195640846217E-14,-1.66321791214608E-16,
1.)) ;
#37179=DIRECTION('ref_axis',(0.707106781186672,0.707106781186423,-3.19988744963517E-14)) ;
#37180=DIRECTION('',(4.54195640846217E-14,-1.66321791214608E-16,1.)) ;
#37181=DIRECTION('center_axis',(4.54195640846217E-14,-1.66321791214608E-16,
1.)) ;
#37182=DIRECTION('ref_axis',(0.707106781186672,0.707106781186423,-3.19988744963517E-14)) ;
#37183=DIRECTION('',(4.54195640846217E-14,-1.66321791214608E-16,1.)) ;
#37184=DIRECTION('center_axis',(4.54195640846217E-14,-1.66321791214608E-16,
1.)) ;
#37185=DIRECTION('ref_axis',(0.707106781186672,0.707106781186423,-3.19988744963517E-14)) ;
#37186=DIRECTION('',(4.54195640846217E-14,-1.66321791214608E-16,1.)) ;
#37187=DIRECTION('center_axis',(4.54195640846217E-14,-1.66321791214601E-16,
1.)) ;
#37188=DIRECTION('ref_axis',(-1.89547329362678E-13,-1.,-1.66321791205992E-16)) ;
#37189=DIRECTION('',(-4.54195640846217E-14,1.66321791214602E-16,-1.)) ;
#37190=DIRECTION('',(4.54195640846217E-14,-1.66321791214602E-16,1.)) ;
#37191=DIRECTION('center_axis',(1.,-1.75658099177411E-13,-4.54195640846217E-14)) ;
#37192=DIRECTION('ref_axis',(-4.54195640846217E-14,1.66321791214601E-16,
-1.)) ;
#37193=DIRECTION('',(4.54195640846217E-14,-1.66321791214602E-16,1.)) ;
#37194=DIRECTION('center_axis',(4.54195640846217E-14,-1.66321791214601E-16,
1.)) ;
#37195=DIRECTION('ref_axis',(1.75658099177411E-13,1.,1.66321791206623E-16)) ;
#37196=DIRECTION('',(-4.54195640846217E-14,1.66321791214602E-16,-1.)) ;
#37197=DIRECTION('center_axis',(-1.,1.75658099177411E-13,4.54195640846217E-14)) ;
#37198=DIRECTION('ref_axis',(4.54195640846217E-14,-1.66321791214601E-16,
1.)) ;
#37199=DIRECTION('center_axis',(4.54195640846217E-14,-1.66321791214601E-16,
1.)) ;
#37200=DIRECTION('ref_axis',(1.75658099177411E-13,1.,1.66321791206623E-16)) ;
#37201=DIRECTION('',(-4.54195640846217E-14,1.66321791214602E-16,-1.)) ;
#37202=DIRECTION('',(4.54195640846217E-14,-1.66321791214602E-16,1.)) ;
#37203=DIRECTION('center_axis',(-1.,1.75658099177411E-13,4.54195640846217E-14)) ;
#37204=DIRECTION('ref_axis',(4.54195640846217E-14,-1.66321791214601E-16,
1.)) ;
#37205=DIRECTION('',(4.54195640846217E-14,-1.66321791214602E-16,1.)) ;
#37206=DIRECTION('center_axis',(4.54195640846217E-14,-1.66321791214601E-16,
1.)) ;
#37207=DIRECTION('ref_axis',(-1.66010601240624E-13,-1.,-1.66321791207061E-16)) ;
#37208=DIRECTION('',(-4.54195640846217E-14,1.66321791214602E-16,-1.)) ;
#37209=DIRECTION('center_axis',(1.,-1.75658099177411E-13,-4.54195640846217E-14)) ;
#37210=DIRECTION('ref_axis',(-4.54195640846217E-14,1.66321791214601E-16,
-1.)) ;
#37211=DIRECTION('center_axis',(4.54195640846217E-14,-1.66321791214601E-16,
1.)) ;
#37212=DIRECTION('ref_axis',(-1.89547329362678E-13,-1.,-1.66321791205992E-16)) ;
#37213=DIRECTION('',(-4.54195640846217E-14,1.66321791214602E-16,-1.)) ;
#37214=DIRECTION('',(4.54195640846217E-14,-1.66321791214602E-16,1.)) ;
#37215=DIRECTION('center_axis',(1.,-1.75658099177411E-13,-4.54195640846217E-14)) ;
#37216=DIRECTION('ref_axis',(-4.54195640846217E-14,1.66321791214601E-16,
-1.)) ;
#37217=DIRECTION('',(4.54195640846217E-14,-1.66321791214602E-16,1.)) ;
#37218=DIRECTION('center_axis',(4.54195640846217E-14,-1.66321791214601E-16,
1.)) ;
#37219=DIRECTION('ref_axis',(1.75658099177411E-13,1.,1.66321791206623E-16)) ;
#37220=DIRECTION('',(-4.54195640846217E-14,1.66321791214602E-16,-1.)) ;
#37221=DIRECTION('center_axis',(-1.,1.75658099177411E-13,4.54195640846217E-14)) ;
#37222=DIRECTION('ref_axis',(4.54195640846217E-14,-1.66321791214601E-16,
1.)) ;
#37223=DIRECTION('center_axis',(4.54195640846217E-14,-1.66321791214601E-16,
1.)) ;
#37224=DIRECTION('ref_axis',(-1.66010601240624E-13,-1.,-1.66321791207061E-16)) ;
#37225=DIRECTION('',(-4.54195640846217E-14,1.66321791214602E-16,-1.)) ;
#37226=DIRECTION('',(4.54195640846217E-14,-1.66321791214602E-16,1.)) ;
#37227=DIRECTION('center_axis',(1.,-1.75658099177411E-13,-4.54195640846217E-14)) ;
#37228=DIRECTION('ref_axis',(-4.54195640846217E-14,1.66321791214601E-16,
-1.)) ;
#37229=DIRECTION('',(4.54195640846217E-14,-1.66321791214602E-16,1.)) ;
#37230=DIRECTION('center_axis',(4.54195640846217E-14,-1.66321791214601E-16,
1.)) ;
#37231=DIRECTION('ref_axis',(1.75658099177411E-13,1.,1.66321791206623E-16)) ;
#37232=DIRECTION('',(-4.54195640846217E-14,1.66321791214602E-16,-1.)) ;
#37233=DIRECTION('center_axis',(-1.,1.75658099177411E-13,4.54195640846217E-14)) ;
#37234=DIRECTION('ref_axis',(4.54195640846217E-14,-1.66321791214601E-16,
1.)) ;
#37235=DIRECTION('center_axis',(4.54195640846217E-14,-1.66321791214601E-16,
1.)) ;
#37236=DIRECTION('ref_axis',(-1.66010601240624E-13,-1.,-1.66321791207061E-16)) ;
#37237=DIRECTION('',(-4.54195640846217E-14,1.66321791214602E-16,-1.)) ;
#37238=DIRECTION('',(4.54195640846217E-14,-1.66321791214602E-16,1.)) ;
#37239=DIRECTION('center_axis',(1.,-1.75658099177411E-13,-4.54195640846217E-14)) ;
#37240=DIRECTION('ref_axis',(-4.54195640846217E-14,1.66321791214601E-16,
-1.)) ;
#37241=DIRECTION('',(4.54195640846217E-14,-1.66321791214602E-16,1.)) ;
#37242=DIRECTION('center_axis',(4.54195640846217E-14,-1.66321791214601E-16,
1.)) ;
#37243=DIRECTION('ref_axis',(1.75658099177411E-13,1.,1.66321791206623E-16)) ;
#37244=DIRECTION('',(-4.54195640846217E-14,1.66321791214602E-16,-1.)) ;
#37245=DIRECTION('center_axis',(-1.,1.75658099177411E-13,4.54195640846217E-14)) ;
#37246=DIRECTION('ref_axis',(4.54195640846217E-14,-1.66321791214601E-16,
1.)) ;
#37247=DIRECTION('center_axis',(4.54195640846217E-14,-1.66321791214601E-16,
1.)) ;
#37248=DIRECTION('ref_axis',(-1.89547329362678E-13,-1.,-1.66321791205992E-16)) ;
#37249=DIRECTION('',(-4.54195640846217E-14,1.66321791214602E-16,-1.)) ;
#37250=DIRECTION('',(4.54195640846217E-14,-1.66321791214602E-16,1.)) ;
#37251=DIRECTION('center_axis',(1.,-1.75658099177411E-13,-4.54195640846217E-14)) ;
#37252=DIRECTION('ref_axis',(-4.54195640846217E-14,1.66321791214601E-16,
-1.)) ;
#37253=DIRECTION('',(4.54195640846217E-14,-1.66321791214602E-16,1.)) ;
#37254=DIRECTION('center_axis',(4.54195640846217E-14,-1.66321791214601E-16,
1.)) ;
#37255=DIRECTION('ref_axis',(1.75658099177411E-13,1.,1.66321791206623E-16)) ;
#37256=DIRECTION('',(-4.54195640846217E-14,1.66321791214602E-16,-1.)) ;
#37257=DIRECTION('center_axis',(-1.,1.75658099177411E-13,4.54195640846217E-14)) ;
#37258=DIRECTION('ref_axis',(4.54195640846217E-14,-1.66321791214601E-16,
1.)) ;
#37259=DIRECTION('center_axis',(-1.75658099177411E-13,-1.,-1.66321791206623E-16)) ;
#37260=DIRECTION('ref_axis',(1.,-1.75658099177411E-13,-4.54195640846217E-14)) ;
#37261=DIRECTION('',(1.75658099177411E-13,1.,1.66321791206623E-16)) ;
#37262=DIRECTION('center_axis',(-1.,1.75658099177411E-13,4.54195640846217E-14)) ;
#37263=DIRECTION('ref_axis',(4.54195640846217E-14,-1.66321791214601E-16,
1.)) ;
#37264=DIRECTION('center_axis',(-1.75658099177411E-13,-1.,-1.66321791206623E-16)) ;
#37265=DIRECTION('ref_axis',(0.99999997726804,-1.75658059720777E-13,-0.000213222701069828)) ;
#37266=DIRECTION('',(-1.75658099177411E-13,-1.,-1.66321791206623E-16)) ;
#37267=DIRECTION('center_axis',(1.08955953009724E-14,-4.58309287791692E-15,
1.)) ;
#37268=DIRECTION('ref_axis',(-0.866025403784527,-0.499999999999848,7.14431588103965E-15)) ;
#37269=DIRECTION('center_axis',(4.9836335171324E-14,-3.46902905748639E-14,
1.)) ;
#37270=DIRECTION('ref_axis',(0.499999999999848,-0.866025403784527,-5.49608404881535E-14)) ;
#37271=DIRECTION('center_axis',(7.99435328682709E-14,4.25044929548771E-15,
1.)) ;
#37272=DIRECTION('ref_axis',(0.866025403784527,0.499999999999848,-7.13583549799491E-14)) ;
#37273=DIRECTION('center_axis',(-1.03934083530628E-14,-3.21183541046639E-14,
1.)) ;
#37274=DIRECTION('ref_axis',(-0.848313848782009,0.529493733640593,8.18959499131937E-15)) ;
#37275=DIRECTION('',(2.48321689126043E-13,-3.16343365850263E-14,-1.)) ;
#37276=DIRECTION('',(-5.79112402932487E-14,7.00367420686418E-14,-1.)) ;
#37277=DIRECTION('center_axis',(1.30601282495909E-14,-5.57440796960452E-14,
1.)) ;
#37278=DIRECTION('ref_axis',(0.848313848782206,0.529493733640277,1.84370532256005E-14)) ;
#37279=DIRECTION('',(8.69448181549043E-14,1.21772749364003E-13,-1.)) ;
#37280=DIRECTION('',(3.35143206547937E-13,5.99821398094943E-14,1.)) ;
#37281=DIRECTION('center_axis',(-2.21832942445859E-16,-4.54750752358529E-14,
1.)) ;
#37282=DIRECTION('ref_axis',(-1.75780563857328E-13,-1.,-4.54750752358529E-14)) ;
#37283=DIRECTION('center_axis',(-2.21832942445859E-16,-4.54750752358529E-14,
1.)) ;
#37284=DIRECTION('ref_axis',(-1.75780563857328E-13,-1.,-4.54750752358529E-14)) ;
#37285=DIRECTION('center_axis',(7.7371596398071E-14,-5.59792942288991E-14,
1.)) ;
#37286=DIRECTION('ref_axis',(-0.529493733640591,-0.84831384878201,-6.52023508487044E-15)) ;
#37287=DIRECTION('',(-1.36189057083808E-14,2.93907575001879E-13,-1.)) ;
#37288=DIRECTION('',(-1.15289984362049E-13,-1.23253544174125E-14,-1.)) ;
#37289=DIRECTION('center_axis',(1.00997321989452E-13,-3.25257576262454E-14,
1.)) ;
#37290=DIRECTION('ref_axis',(-0.52949373364028,0.848313848782204,8.10694997443418E-14)) ;
#37291=DIRECTION('',(-1.6702599165741E-13,1.32530704030741E-13,-1.)) ;
#37292=DIRECTION('',(-1.47288975160872E-14,2.895573206721E-13,1.)) ;
#37293=DIRECTION('center_axis',(9.072831752926E-14,-4.58077188182821E-14,
1.)) ;
#37294=DIRECTION('ref_axis',(1.,-1.75841796197283E-13,-9.07283175292681E-14)) ;
#37295=DIRECTION('center_axis',(9.072831752926E-14,-4.58077188182821E-14,
1.)) ;
#37296=DIRECTION('ref_axis',(1.,-1.75841796197283E-13,-9.07283175292681E-14)) ;
#37297=DIRECTION('center_axis',(1.01232536522306E-13,3.17857105222347E-14,
1.)) ;
#37298=DIRECTION('ref_axis',(0.848313848782008,-0.529493733640594,-6.90466281383654E-14)) ;
#37299=DIRECTION('',(-3.39160817295286E-13,3.19669801674555E-14,-1.)) ;
#37300=DIRECTION('',(-3.29278878759946E-14,-6.97040984862126E-14,-1.)) ;
#37301=DIRECTION('center_axis',(7.77789999196525E-14,5.5411436113616E-14,
1.)) ;
#37302=DIRECTION('ref_axis',(-0.848313848782201,-0.529493733640285,9.53210109704396E-14)) ;
#37303=DIRECTION('',(-1.77783946324148E-13,-1.21440105781574E-13,-1.)) ;
#37304=DIRECTION('',(-2.44304078378693E-13,-6.03147833919235E-14,1.)) ;
#37305=DIRECTION('center_axis',(9.10609611116892E-14,4.51424316534237E-14,
1.)) ;
#37306=DIRECTION('ref_axis',(1.75903028537238E-13,1.,-4.51424316534397E-14)) ;
#37307=DIRECTION('center_axis',(9.10609611116892E-14,4.51424316534237E-14,
1.)) ;
#37308=DIRECTION('ref_axis',(1.75903028537238E-13,1.,-4.51424316534397E-14)) ;
#46348=CARTESIAN_POINT('',(0.,0.,0.)) ;
#46349=CARTESIAN_POINT('Origin',(209.138527625422,615.860565160531,-20.372160171761)) ;
#46350=CARTESIAN_POINT('',(196.738527625422,616.110565160533,-20.3721601717605)) ;
#46351=CARTESIAN_POINT('',(196.738527625422,615.860565160533,-20.1221601717605)) ;
#46352=CARTESIAN_POINT('Origin',(196.738527625422,615.860565160533,-20.3721601717605)) ;
#46353=CARTESIAN_POINT('',(0.238527625422233,615.860565160567,-20.1221601717516)) ;
#46354=CARTESIAN_POINT('',(209.138527625422,615.860565160531,-20.122160171761)) ;
#46355=CARTESIAN_POINT('',(0.23852762542226,616.110565160567,-20.3721601717515)) ;
#46356=CARTESIAN_POINT('Origin',(0.238527625422229,615.860565160567,-20.3721601717515)) ;
#46357=CARTESIAN_POINT('',(209.138527625422,616.110565160531,-20.372160171761)) ;
#46358=CARTESIAN_POINT('Origin',(205.888527625422,616.210565160531,-20.1221601717609)) ;
#46359=CARTESIAN_POINT('',(196.738527625403,506.560565160533,-20.1221601717605)) ;
#46360=CARTESIAN_POINT('',(196.738527625422,616.210565160533,-20.1221601717605)) ;
#46361=CARTESIAN_POINT('',(0.238527625403034,506.560565160567,-20.1221601717516)) ;
#46362=CARTESIAN_POINT('',(209.138527625403,506.560565160531,-20.1221601717611)) ;
#46363=CARTESIAN_POINT('',(0.2385276254034,508.710565160567,-20.1221601717516)) ;
#46364=CARTESIAN_POINT('',(0.238527625422229,615.835565160567,-20.1221601717516)) ;
#46365=CARTESIAN_POINT('',(0.238527625421856,613.710565160567,-20.1221601717515)) ;
#46366=CARTESIAN_POINT('',(0.238527625417512,588.710565160567,-20.1221601717516)) ;
#46367=CARTESIAN_POINT('',(0.238527625422229,615.835565160567,-20.1221601717516)) ;
#46368=CARTESIAN_POINT('',(68.1896090740378,536.698209005427,-20.1221601717547)) ;
#46369=CARTESIAN_POINT('',(48.6516101218399,517.160211426462,-20.1221601717564)) ;
#46370=CARTESIAN_POINT('Origin',(44.9784504245142,540.371370334153,-20.1221601717596)) ;
#46371=CARTESIAN_POINT('',(49.433135115108,512.221667239673,-20.1221601717538)) ;
#46372=CARTESIAN_POINT('Ctrl Pts',(49.4331351151386,512.22166723948,-20.1221601717538)) ;
#46373=CARTESIAN_POINT('Ctrl Pts',(49.0637330002203,512.163209431222,-20.122160171973)) ;
#46374=CARTESIAN_POINT('Ctrl Pts',(47.9122384134768,512.229997790623,-20.1221601726336)) ;
#46375=CARTESIAN_POINT('Ctrl Pts',(46.385300085782,513.6230574364,-20.1221601733896)) ;
#46376=CARTESIAN_POINT('Ctrl Pts',(46.5550515020585,516.100143194611,-20.1221601730646)) ;
#46377=CARTESIAN_POINT('Ctrl Pts',(47.91280440288,517.043294655983,-20.1221601721921)) ;
#46378=CARTESIAN_POINT('Ctrl Pts',(48.6516084909445,517.16021116837,-20.1221601717537)) ;
#46379=CARTESIAN_POINT('',(73.1281534675486,535.916685318467,-20.1221601717549)) ;
#46380=CARTESIAN_POINT('Origin',(44.9784504245142,540.371370334153,-20.1221601717536)) ;
#46381=CARTESIAN_POINT('Origin',(70.6588812706952,536.307447161957,-20.1221601717603)) ;
#46382=CARTESIAN_POINT('',(16.8287456930678,535.916695987763,-20.1221601717523)) ;
#46383=CARTESIAN_POINT('',(21.7672748307833,536.698316071089,-20.122160171752)) ;
#46384=CARTESIAN_POINT('Ctrl Pts',(16.8287456930845,535.916695987658,-20.1221601717523)) ;
#46385=CARTESIAN_POINT('Ctrl Pts',(16.7702887385344,536.286093587143,-20.1221601717711)) ;
#46386=CARTESIAN_POINT('Ctrl Pts',(16.8370747519972,537.437573131114,-20.1221601718281)) ;
#46387=CARTESIAN_POINT('Ctrl Pts',(18.2300981773897,538.964503729432,-20.1221601718931)) ;
#46388=CARTESIAN_POINT('Ctrl Pts',(20.7071515274629,538.7948086885,-20.1221601718654)) ;
#46389=CARTESIAN_POINT('Ctrl Pts',(21.6503315190709,537.437106616922,-20.1221601717903)) ;
#46390=CARTESIAN_POINT('Ctrl Pts',(21.7672748296711,536.698316071321,-20.1221601717526)) ;
#46391=CARTESIAN_POINT('',(40.523765408828,512.221667291119,-20.1221601717534)) ;
#46392=CARTESIAN_POINT('Origin',(44.9784504245142,540.371370334153,-20.1221601717536)) ;
#46393=CARTESIAN_POINT('',(41.3052890957878,517.16021168463,-20.1221601717534)) ;
#46394=CARTESIAN_POINT('Origin',(40.9145272523186,514.690939487972,-20.1221601717542)) ;
#46395=CARTESIAN_POINT('Origin',(44.9784504245141,540.371370334153,-20.1221601717517)) ;
#46396=CARTESIAN_POINT('',(40.5237715662164,568.521074351592,-20.1221601670422)) ;
#46397=CARTESIAN_POINT('',(41.3053508856094,563.582538762398,-20.1221601670332)) ;
#46398=CARTESIAN_POINT('Origin',(40.9145328695252,566.051802069454,-20.1221601615182)) ;
#46399=CARTESIAN_POINT('',(16.8287473814797,544.826055349839,-20.1221601717523)) ;
#46400=CARTESIAN_POINT('Origin',(44.9784504245142,540.371370334153,-20.1221601717536)) ;
#46401=CARTESIAN_POINT('',(21.7672917749906,544.04453166288,-20.1221601717525)) ;
#46402=CARTESIAN_POINT('Origin',(19.2980195783332,544.435293506349,-20.1221601717457)) ;
#46403=CARTESIAN_POINT('Origin',(44.9784504245142,540.371370334153,-20.1221601717476)) ;
#46404=CARTESIAN_POINT('',(31.8295857683878,532.164217462742,-20.122160171753)) ;
#46405=CARTESIAN_POINT('',(31.8295857683906,548.578523205569,-20.122160171753)) ;
#46406=CARTESIAN_POINT('Origin',(44.978450424514,540.371370334153,-20.1221601717575)) ;
#46407=CARTESIAN_POINT('',(26.7397026756955,551.755485607418,-20.1221601717528)) ;
#46408=CARTESIAN_POINT('Origin',(29.284644222043,550.167004406493,-20.1221601717549)) ;
#46409=CARTESIAN_POINT('',(26.7397026756915,528.987255060894,-20.1221601717528)) ;
#46410=CARTESIAN_POINT('Origin',(44.978450424514,540.371370334153,-20.1221601717575)) ;
#46411=CARTESIAN_POINT('Origin',(29.2846442220397,530.575736261818,-20.1221601717601)) ;
#46412=CARTESIAN_POINT('',(158.588527625415,572.710565160539,-20.1221601717588)) ;
#46413=CARTESIAN_POINT('',(158.588527625419,594.710565160539,-20.1221601717587)) ;
#46414=CARTESIAN_POINT('',(158.58852762542,605.460565160539,-20.1221601717588)) ;
#46415=CARTESIAN_POINT('',(161.588527625415,572.710565160539,-20.1221601717589)) ;
#46416=CARTESIAN_POINT('Origin',(160.088527625415,572.710565160539,-20.1221601717588)) ;
#46417=CARTESIAN_POINT('',(161.588527625419,594.710565160539,-20.1221601717589)) ;
#46418=CARTESIAN_POINT('',(161.588527625419,594.460565160539,-20.1221601717589)) ;
#46419=CARTESIAN_POINT('Origin',(160.088527625419,594.710565160539,-20.1221601717588)) ;
#46420=CARTESIAN_POINT('',(165.588527625415,572.710565160538,-20.1221601717591)) ;
#46421=CARTESIAN_POINT('',(165.588527625419,594.710565160538,-20.1221601717591)) ;
#46422=CARTESIAN_POINT('',(165.58852762542,605.460565160538,-20.1221601717591)) ;
#46423=CARTESIAN_POINT('',(168.588527625415,572.710565160538,-20.1221601717592)) ;
#46424=CARTESIAN_POINT('Origin',(167.088527625415,572.710565160538,-20.1221601717592)) ;
#46425=CARTESIAN_POINT('',(168.588527625419,594.710565160538,-20.1221601717592)) ;
#46426=CARTESIAN_POINT('',(168.588527625419,594.460565160538,-20.1221601717592)) ;
#46427=CARTESIAN_POINT('Origin',(167.088527625419,594.710565160538,-20.1221601717591)) ;
#46428=CARTESIAN_POINT('',(172.588527625415,572.710565160537,-20.1221601717594)) ;
#46429=CARTESIAN_POINT('',(172.588527625419,594.710565160537,-20.1221601717594)) ;
#46430=CARTESIAN_POINT('',(172.58852762542,605.460565160537,-20.1221601717594)) ;
#46431=CARTESIAN_POINT('',(175.588527625415,572.710565160536,-20.1221601717595)) ;
#46432=CARTESIAN_POINT('Origin',(174.088527625415,572.710565160537,-20.1221601717595)) ;
#46433=CARTESIAN_POINT('',(175.588527625419,594.710565160536,-20.1221601717595)) ;
#46434=CARTESIAN_POINT('',(175.588527625419,594.460565160536,-20.1221601717595)) ;
#46435=CARTESIAN_POINT('Origin',(174.088527625419,594.710565160537,-20.1221601717594)) ;
#46436=CARTESIAN_POINT('',(158.588527625407,527.710565160539,-20.1221601717588)) ;
#46437=CARTESIAN_POINT('',(158.588527625411,549.710565160539,-20.1221601717588)) ;
#46438=CARTESIAN_POINT('',(158.588527625417,582.960565160539,-20.1221601717588)) ;
#46439=CARTESIAN_POINT('',(161.588527625407,527.710565160539,-20.1221601717589)) ;
#46440=CARTESIAN_POINT('Origin',(160.088527625407,527.710565160539,-20.1221601717588)) ;
#46441=CARTESIAN_POINT('',(161.588527625411,549.710565160539,-20.1221601717589)) ;
#46442=CARTESIAN_POINT('',(161.588527625415,571.960565160539,-20.1221601717589)) ;
#46443=CARTESIAN_POINT('Origin',(160.088527625411,549.710565160539,-20.1221601717588)) ;
#46444=CARTESIAN_POINT('',(168.588527625411,549.710565160538,-20.1221601717592)) ;
#46445=CARTESIAN_POINT('',(168.588527625407,527.710565160538,-20.1221601717592)) ;
#46446=CARTESIAN_POINT('',(168.588527625415,571.960565160538,-20.1221601717592)) ;
#46447=CARTESIAN_POINT('',(165.588527625411,549.710565160538,-20.1221601717591)) ;
#46448=CARTESIAN_POINT('Origin',(167.088527625411,549.710565160538,-20.1221601717592)) ;
#46449=CARTESIAN_POINT('',(165.588527625407,527.710565160538,-20.1221601717591)) ;
#46450=CARTESIAN_POINT('',(165.588527625416,582.960565160538,-20.1221601717591)) ;
#46451=CARTESIAN_POINT('Origin',(167.088527625407,527.710565160538,-20.1221601717592)) ;
#46452=CARTESIAN_POINT('',(172.588527625407,527.710565160537,-20.1221601717594)) ;
#46453=CARTESIAN_POINT('',(172.588527625411,549.710565160537,-20.1221601717594)) ;
#46454=CARTESIAN_POINT('',(172.588527625417,582.960565160537,-20.1221601717594)) ;
#46455=CARTESIAN_POINT('',(175.588527625407,527.710565160536,-20.1221601717595)) ;
#46456=CARTESIAN_POINT('Origin',(174.088527625407,527.710565160537,-20.1221601717595)) ;
#46457=CARTESIAN_POINT('',(175.588527625411,549.710565160536,-20.1221601717595)) ;
#46458=CARTESIAN_POINT('',(175.588527625415,571.960565160536,-20.1221601717595)) ;
#46459=CARTESIAN_POINT('Origin',(174.088527625411,549.710565160537,-20.1221601717595)) ;
#46460=CARTESIAN_POINT('',(67.9918523583144,515.591787908231,-20.1221601717546)) ;
#46461=CARTESIAN_POINT('Origin',(69.8918523583194,515.59178790823,-20.1221601717547)) ;
#46462=CARTESIAN_POINT('',(17.9918523583232,565.591787908239,-20.1221601717524)) ;
#46463=CARTESIAN_POINT('Origin',(19.8918523583282,565.591787908239,-20.1221601717525)) ;
#46464=CARTESIAN_POINT('',(43.5689387445144,545.577405470032,-20.1221601717535)) ;
#46465=CARTESIAN_POINT('Origin',(44.9831523068878,546.991619032404,-20.1221601717536)) ;
#46466=CARTESIAN_POINT('',(37.0744829388653,539.087651546757,-20.1221601717532)) ;
#46467=CARTESIAN_POINT('Origin',(38.4886965012387,540.50186510913,-20.1221601717533)) ;
#46468=CARTESIAN_POINT('',(43.5642368621325,532.593195741101,-20.1221601717535)) ;
#46469=CARTESIAN_POINT('Origin',(44.9784504245058,534.007409303474,-20.1221601717536)) ;
#46470=CARTESIAN_POINT('',(50.0586926677957,539.082949664375,-20.1221601717538)) ;
#46471=CARTESIAN_POINT('Origin',(51.472906230169,540.497163226748,-20.1221601717539)) ;
#46472=CARTESIAN_POINT('',(33.5943351512492,522.132622585335,-20.1221601717531)) ;
#46473=CARTESIAN_POINT('',(36.7712975530989,527.22250567803,-20.1221601717532)) ;
#46474=CARTESIAN_POINT('Origin',(35.1828163521739,524.677564131682,-20.1221601717657)) ;
#46475=CARTESIAN_POINT('',(56.3625656977731,522.13262258533,-20.1221601717541)) ;
#46476=CARTESIAN_POINT('Origin',(44.9784504245142,540.371370334153,-20.1221601717645)) ;
#46477=CARTESIAN_POINT('',(53.1856032959252,527.222505678027,-20.122160171754)) ;
#46478=CARTESIAN_POINT('Origin',(54.774084496849,524.677564131679,-20.1221601717641)) ;
#46479=CARTESIAN_POINT('Origin',(44.9784504245142,540.371370334153,-20.1221601717645)) ;
#46480=CARTESIAN_POINT('',(63.2171981733329,528.987255060888,-20.1221601717544)) ;
#46481=CARTESIAN_POINT('',(58.1273150806378,532.164217462738,-20.1221601717542)) ;
#46482=CARTESIAN_POINT('Origin',(60.6722566269853,530.575736261813,-20.1221601717544)) ;
#46483=CARTESIAN_POINT('',(63.2171981733369,551.755485607412,-20.1221601717544)) ;
#46484=CARTESIAN_POINT('Origin',(44.9784504245143,540.371370334153,-20.1221601717496)) ;
#46485=CARTESIAN_POINT('',(58.1273150806405,548.578523205564,-20.1221601717542)) ;
#46486=CARTESIAN_POINT('Origin',(60.6722566269887,550.167004406488,-20.1221601717483)) ;
#46487=CARTESIAN_POINT('Origin',(44.9784504245143,540.371370334153,-20.1221601717496)) ;
#46488=CARTESIAN_POINT('',(56.3625656977793,558.610118082972,-20.1221601717541)) ;
#46489=CARTESIAN_POINT('',(53.1856032959296,553.520234990277,-20.122160171754)) ;
#46490=CARTESIAN_POINT('Origin',(54.7740844968544,556.065176536624,-20.1221601717435)) ;
#46491=CARTESIAN_POINT('',(33.5943351512553,558.610118082976,-20.1221601717531)) ;
#46492=CARTESIAN_POINT('Origin',(44.9784504245142,540.371370334153,-20.1221601717427)) ;
#46493=CARTESIAN_POINT('',(36.7712975531032,553.52023499028,-20.1221601717532)) ;
#46494=CARTESIAN_POINT('Origin',(35.1828163521793,556.065176536628,-20.1221601717442)) ;
#46495=CARTESIAN_POINT('Origin',(44.9784504245142,540.371370334153,-20.1221601717427)) ;
#46496=CARTESIAN_POINT('',(48.6516117532405,563.582528983677,-20.1221601717538)) ;
#46497=CARTESIAN_POINT('',(68.189609074102,544.044531662882,-20.1221601728767)) ;
#46498=CARTESIAN_POINT('Origin',(44.9784504245142,540.371370334153,-20.1221601717555)) ;
#46499=CARTESIAN_POINT('',(73.1281535186845,544.826055026706,-20.1221601728761)) ;
#46500=CARTESIAN_POINT('Origin',(70.6588813175355,544.435293211616,-20.1221601742775)) ;
#46501=CARTESIAN_POINT('',(49.4331354401999,568.521073377188,-20.1221601717538)) ;
#46502=CARTESIAN_POINT('Origin',(44.9784504245142,540.371370334153,-20.1221601717536)) ;
#46503=CARTESIAN_POINT('Origin',(49.0423735967098,566.051801180334,-20.1221601717518)) ;
#46504=CARTESIAN_POINT('Origin',(0.238527625417501,588.710565160567,-20.3721601717516)) ;
#46505=CARTESIAN_POINT('',(-0.0114723745781272,613.710565160567,-20.3721601717515)) ;
#46506=CARTESIAN_POINT('Origin',(0.238527625421892,613.710565160567,-20.3721601717515)) ;
#46507=CARTESIAN_POINT('',(-0.0114723745965713,508.710565160567,-20.3721601717516)) ;
#46508=CARTESIAN_POINT('Origin',(0.238527625403448,508.710565160567,-20.3721601717516)) ;
#46509=CARTESIAN_POINT('',(-0.0114723745825186,588.710565160567,-20.3721601717515)) ;
#46510=CARTESIAN_POINT('Origin',(209.138527625403,506.560565160531,-20.3721601717611)) ;
#46511=CARTESIAN_POINT('',(196.738527625403,506.310565160533,-20.3721601717605)) ;
#46512=CARTESIAN_POINT('Origin',(196.738527625403,506.560565160533,-20.3721601717605)) ;
#46513=CARTESIAN_POINT('',(0.238527625402987,506.310565160567,-20.3721601717516)) ;
#46514=CARTESIAN_POINT('',(209.138527625403,506.310565160531,-20.3721601717611)) ;
#46515=CARTESIAN_POINT('Origin',(0.238527625403044,506.560565160567,-20.3721601717516)) ;
#46516=CARTESIAN_POINT('Origin',(212.388527625401,506.31056516053,-69.5221601717612)) ;
#46517=CARTESIAN_POINT('',(196.738527625403,506.310565160533,-23.5221601717605)) ;
#46518=CARTESIAN_POINT('',(196.738527625402,506.310565160533,-44.5221601717605)) ;
#46519=CARTESIAN_POINT('',(196.238527625403,506.310565160533,-24.0221601717605)) ;
#46520=CARTESIAN_POINT('Origin',(196.238527625403,506.310565160533,-23.5221601717605)) ;
#46521=CARTESIAN_POINT('',(193.388264603403,506.310565160533,-24.0221601717603)) ;
#46522=CARTESIAN_POINT('',(203.313527625403,506.310565160532,-24.0221601717608)) ;
#46523=CARTESIAN_POINT('',(192.388264603403,506.310565160534,-25.0221601717604)) ;
#46524=CARTESIAN_POINT('Origin',(193.388264603403,506.310565160533,-25.0221601717604)) ;
#46525=CARTESIAN_POINT('',(192.388264603403,506.310565160534,-27.5221601717603)) ;
#46526=CARTESIAN_POINT('',(192.388264603403,506.310565160534,-46.7721601717608)) ;
#46527=CARTESIAN_POINT('',(191.388264603403,506.310565160534,-28.5221601717603)) ;
#46528=CARTESIAN_POINT('Origin',(191.388264603403,506.310565160534,-27.5221601717603)) ;
#46529=CARTESIAN_POINT('',(183.388264603403,506.310565160535,-28.5221601717599)) ;
#46530=CARTESIAN_POINT('',(205.813527625403,506.310565160531,-28.5221601717609)) ;
#46531=CARTESIAN_POINT('',(182.388264603403,506.310565160535,-27.5221601717599)) ;
#46532=CARTESIAN_POINT('Origin',(183.388264603403,506.310565160535,-27.5221601717599)) ;
#46533=CARTESIAN_POINT('',(182.388264603403,506.310565160535,-25.0221601717598)) ;
#46534=CARTESIAN_POINT('',(182.388264603403,506.310565160535,-49.0221601717605)) ;
#46535=CARTESIAN_POINT('',(181.388264603403,506.310565160536,-24.0221601717598)) ;
#46536=CARTESIAN_POINT('Origin',(181.388264603403,506.310565160535,-25.0221601717598)) ;
#46537=CARTESIAN_POINT('',(12.4885276254027,506.310565160565,-24.0221601717521)) ;
#46538=CARTESIAN_POINT('',(197.388396114403,506.310565160533,-24.0221601717605)) ;
#46539=CARTESIAN_POINT('',(11.4885276254026,506.310565160565,-25.0221601717521)) ;
#46540=CARTESIAN_POINT('Origin',(12.4885276254026,506.310565160565,-25.0221601717521)) ;
#46541=CARTESIAN_POINT('',(11.4885276254026,506.310565160565,-27.522160171752)) ;
#46542=CARTESIAN_POINT('',(11.4885276254026,506.310565160565,-46.7721601717567)) ;
#46543=CARTESIAN_POINT('',(10.4885276254026,506.310565160566,-28.522160171752)) ;
#46544=CARTESIAN_POINT('Origin',(10.4885276254026,506.310565160565,-27.522160171752)) ;
#46545=CARTESIAN_POINT('',(1.2385276254026,506.310565160567,-28.5221601717516)) ;
#46546=CARTESIAN_POINT('',(205.813527625403,506.310565160531,-28.5221601717609)) ;
#46547=CARTESIAN_POINT('',(0.238527625402662,506.310565160567,-27.5221601717516)) ;
#46548=CARTESIAN_POINT('Origin',(1.23852762540266,506.310565160567,-27.5221601717516)) ;
#46549=CARTESIAN_POINT('',(0.23852762540189,506.310565160567,-44.5221601717516)) ;
#46550=CARTESIAN_POINT('',(188.638264603403,506.310565160534,-24.0203292412001)) ;
#46551=CARTESIAN_POINT('Origin',(187.388264603403,506.310565160534,-24.0203292412001)) ;
#46552=CARTESIAN_POINT('',(7.73852762540263,506.310565160566,-24.0221601717538)) ;
#46553=CARTESIAN_POINT('Origin',(6.48852762540263,506.310565160566,-24.0221601717538)) ;
#46554=CARTESIAN_POINT('Origin',(155.388527625422,615.96056516054,-20.2721601717586)) ;
#46555=CARTESIAN_POINT('',(0.23852762542239,616.710565160567,-20.2721601717516)) ;
#46556=CARTESIAN_POINT('',(0.238527625422287,615.960565160567,-19.5221601717516)) ;
#46557=CARTESIAN_POINT('Origin',(0.238527625422247,615.960565160567,-20.2721601717516)) ;
#46558=CARTESIAN_POINT('',(196.738527625422,615.960565160533,-19.5221601717605)) ;
#46559=CARTESIAN_POINT('',(155.388527625422,615.96056516054,-19.5221601717586)) ;
#46560=CARTESIAN_POINT('',(196.738527625422,616.710565160533,-20.2721601717605)) ;
#46561=CARTESIAN_POINT('Origin',(196.738527625422,615.960565160533,-20.2721601717605)) ;
#46562=CARTESIAN_POINT('',(155.388527625422,616.71056516054,-20.2721601717586)) ;
#46563=CARTESIAN_POINT('Origin',(0.238527625422194,615.460565160567,-19.5221601717516)) ;
#46564=CARTESIAN_POINT('',(0.238527625422061,616.710565160567,-27.5221601717515)) ;
#46565=CARTESIAN_POINT('',(0.238527625421743,616.710565160567,-34.5221601717516)) ;
#46566=CARTESIAN_POINT('',(0.238527625421935,616.110565160567,-27.5221601717515)) ;
#46567=CARTESIAN_POINT('',(0.23852762542194,616.085565160567,-27.5221601717515)) ;
#46568=CARTESIAN_POINT('',(0.238527625421163,616.110565160567,-44.5221601717516)) ;
#46569=CARTESIAN_POINT('',(0.238527625421886,613.710565160567,-19.5221601717516)) ;
#46570=CARTESIAN_POINT('',(0.238527625421886,613.710565160567,-19.5221601717516)) ;
#46571=CARTESIAN_POINT('',(0.238527625422265,615.835565160567,-19.5221601717516)) ;
#46572=CARTESIAN_POINT('Origin',(104.888527625422,616.710565160549,-34.4971601717606)) ;
#46573=CARTESIAN_POINT('',(196.738527625422,616.710565160533,-23.5221601717605)) ;
#46574=CARTESIAN_POINT('',(196.738527625422,616.710565160533,-34.5221601717605)) ;
#46575=CARTESIAN_POINT('',(196.238527625422,616.710565160533,-24.0221601717605)) ;
#46576=CARTESIAN_POINT('Origin',(196.238527625422,616.710565160533,-23.5221601717605)) ;
#46577=CARTESIAN_POINT('',(193.388264603422,616.710565160533,-24.0221601717603)) ;
#46578=CARTESIAN_POINT('',(149.563527625422,616.710565160541,-24.0221601717583)) ;
#46579=CARTESIAN_POINT('',(192.388264603422,616.710565160533,-25.0221601717603)) ;
#46580=CARTESIAN_POINT('Origin',(193.388264603422,616.710565160533,-25.0221601717603)) ;
#46581=CARTESIAN_POINT('',(192.388264603422,616.710565160533,-27.5221601717598)) ;
#46582=CARTESIAN_POINT('',(192.388264603422,616.710565160533,-28.7221601717598)) ;
#46583=CARTESIAN_POINT('',(191.388264603422,616.710565160534,-28.5221601717598)) ;
#46584=CARTESIAN_POINT('Origin',(191.388264603422,616.710565160532,-27.5221601717598)) ;
#46585=CARTESIAN_POINT('',(183.388264603422,616.710565160535,-28.5221601717598)) ;
#46586=CARTESIAN_POINT('',(143.638396114422,616.710565160542,-28.5221601717598)) ;
#46587=CARTESIAN_POINT('',(182.388264603422,616.710565160535,-27.5221601717598)) ;
#46588=CARTESIAN_POINT('Origin',(183.388264603422,616.710565160534,-27.5221601717598)) ;
#46589=CARTESIAN_POINT('',(182.388264603422,616.710565160535,-25.0221601717598)) ;
#46590=CARTESIAN_POINT('',(182.388264603422,616.710565160535,-19.5221601717598)) ;
#46591=CARTESIAN_POINT('',(181.388264603422,616.710565160535,-24.0221601717598)) ;
#46592=CARTESIAN_POINT('Origin',(181.388264603422,616.710565160534,-25.0221601717598)) ;
#46593=CARTESIAN_POINT('',(12.4885276254221,616.710565160565,-24.0221601717521)) ;
#46594=CARTESIAN_POINT('',(152.063527625422,616.71056516054,-24.0221601717585)) ;
#46595=CARTESIAN_POINT('',(11.488527625422,616.710565160565,-25.0221601717521)) ;
#46596=CARTESIAN_POINT('Origin',(12.488527625422,616.710565160565,-25.0221601717521)) ;
#46597=CARTESIAN_POINT('',(11.488527625422,616.710565160565,-27.5221601717516)) ;
#46598=CARTESIAN_POINT('',(11.488527625422,616.710565160565,-19.5221601717561)) ;
#46599=CARTESIAN_POINT('',(10.488527625422,616.710565160565,-28.5221603701969)) ;
#46600=CARTESIAN_POINT('Origin',(10.488527625422,616.710565160565,-27.5221601717516)) ;
#46601=CARTESIAN_POINT('',(1.23852762542205,616.710565160567,-28.5221603701968)) ;
#46602=CARTESIAN_POINT('',(152.063527625422,616.71056516054,-28.522160767094)) ;
#46603=CARTESIAN_POINT('Origin',(1.23852762542205,616.710565160567,-27.5221601717516)) ;
#46604=CARTESIAN_POINT('',(186.138264631837,616.710565160535,-24.0200627128237)) ;
#46605=CARTESIAN_POINT('Origin',(187.388264603422,616.710565160534,-24.0203292412001)) ;
#46606=CARTESIAN_POINT('',(7.73852762542202,616.710565160566,-24.0221601717538)) ;
#46607=CARTESIAN_POINT('Origin',(6.48852762542202,616.710565160566,-24.0221601717538)) ;
#46608=CARTESIAN_POINT('Origin',(209.138527625403,506.460565160531,-20.2721601717611)) ;
#46609=CARTESIAN_POINT('',(196.738527625403,505.710565160533,-20.2721601717605)) ;
#46610=CARTESIAN_POINT('',(196.738527625403,506.460565160533,-19.5221601717605)) ;
#46611=CARTESIAN_POINT('Origin',(196.738527625403,506.460565160533,-20.2721601717605)) ;
#46612=CARTESIAN_POINT('',(0.238527625403083,506.460565160567,-19.5221601717516)) ;
#46613=CARTESIAN_POINT('',(209.138527625403,506.460565160531,-19.5221601717611)) ;
#46614=CARTESIAN_POINT('',(0.238527625402882,505.710565160567,-20.2721601717516)) ;
#46615=CARTESIAN_POINT('Origin',(0.238527625403009,506.460565160567,-20.2721601717516)) ;
#46616=CARTESIAN_POINT('',(209.138527625403,505.710565160531,-20.2721601717611)) ;
#46617=CARTESIAN_POINT('Origin',(196.738527625422,616.210565160533,-19.5221601717605)) ;
#46618=CARTESIAN_POINT('',(196.738527625403,505.710565160533,-23.5221601717605)) ;
#46619=CARTESIAN_POINT('',(196.738527625403,505.710565160533,-9.5221601717605)) ;
#46620=CARTESIAN_POINT('',(196.738527625422,616.460565160533,-23.5221601717605)) ;
#46621=CARTESIAN_POINT('',(196.738527625403,506.560565160533,-19.5221601717605)) ;
#46622=CARTESIAN_POINT('',(196.738527625403,506.560565160533,-19.5221601717605)) ;
#46623=CARTESIAN_POINT('',(196.738527625422,616.210565160533,-19.5221601717605)) ;
#46624=CARTESIAN_POINT('Origin',(212.388527625404,505.71056516053,0.477839828238782)) ;
#46625=CARTESIAN_POINT('',(0.238527625402582,505.710565160567,-27.5221601717516)) ;
#46626=CARTESIAN_POINT('',(0.238527625403371,505.710565160567,-9.52216017175159)) ;
#46627=CARTESIAN_POINT('',(1.23852762540249,505.710565160567,-28.5221601717516)) ;
#46628=CARTESIAN_POINT('Origin',(1.23852762540256,505.710565160567,-27.5221601717516)) ;
#46629=CARTESIAN_POINT('',(10.4885276254025,505.710565160566,-28.522160171752)) ;
#46630=CARTESIAN_POINT('',(205.813527625403,505.710565160531,-28.5221601717609)) ;
#46631=CARTESIAN_POINT('',(11.4885276254025,505.710565160565,-27.522160171752)) ;
#46632=CARTESIAN_POINT('Origin',(10.4885276254025,505.710565160565,-27.522160171752)) ;
#46633=CARTESIAN_POINT('',(11.4885276254025,505.710565160565,-25.0221601717521)) ;
#46634=CARTESIAN_POINT('',(11.4885276254025,505.710565160565,-11.7721601717567)) ;
#46635=CARTESIAN_POINT('',(12.4885276254026,505.710565160565,-24.0221601717521)) ;
#46636=CARTESIAN_POINT('Origin',(12.4885276254025,505.710565160564,-25.0221601717521)) ;
#46637=CARTESIAN_POINT('',(181.388264603403,505.710565160536,-24.0221601717598)) ;
#46638=CARTESIAN_POINT('',(197.388396114403,505.710565160533,-24.0221601717605)) ;
#46639=CARTESIAN_POINT('',(182.388264603403,505.710565160535,-25.0221601717598)) ;
#46640=CARTESIAN_POINT('Origin',(181.388264603403,505.710565160535,-25.0221601717598)) ;
#46641=CARTESIAN_POINT('',(182.388264603403,505.710565160535,-27.5221601717599)) ;
#46642=CARTESIAN_POINT('',(182.388264603403,505.710565160535,-14.0221601717605)) ;
#46643=CARTESIAN_POINT('',(183.388264603403,505.710565160535,-28.5221601717599)) ;
#46644=CARTESIAN_POINT('Origin',(183.388264603403,505.710565160535,-27.5221601717599)) ;
#46645=CARTESIAN_POINT('',(191.388264603403,505.710565160534,-28.5221601717603)) ;
#46646=CARTESIAN_POINT('',(205.813527625403,505.710565160531,-28.5221601717609)) ;
#46647=CARTESIAN_POINT('',(192.388264603403,505.710565160534,-27.5221601717603)) ;
#46648=CARTESIAN_POINT('Origin',(191.388264603403,505.710565160534,-27.5221601717603)) ;
#46649=CARTESIAN_POINT('',(192.388264603403,505.710565160534,-25.0221601717603)) ;
#46650=CARTESIAN_POINT('',(192.388264603403,505.710565160534,-11.7721601717608)) ;
#46651=CARTESIAN_POINT('',(193.388264603403,505.710565160533,-24.0221601717603)) ;
#46652=CARTESIAN_POINT('Origin',(193.388264603403,505.710565160533,-25.0221601717604)) ;
#46653=CARTESIAN_POINT('',(196.238527625403,505.710565160533,-24.0221601717605)) ;
#46654=CARTESIAN_POINT('',(203.313527625403,505.710565160532,-24.0221601717608)) ;
#46655=CARTESIAN_POINT('Origin',(196.238527625403,505.710565160533,-23.5221601717605)) ;
#46656=CARTESIAN_POINT('',(188.638264603403,505.710565160534,-24.0203292412001)) ;
#46657=CARTESIAN_POINT('Origin',(187.388264603403,505.710565160534,-24.0203292412001)) ;
#46658=CARTESIAN_POINT('',(7.73852762540252,505.710565160566,-24.0221601717538)) ;
#46659=CARTESIAN_POINT('Origin',(6.48852762540252,505.710565160566,-24.0221601717538)) ;
#46660=CARTESIAN_POINT('Origin',(193.388264603422,616.710565160533,-25.0221601717603)) ;
#46661=CARTESIAN_POINT('',(193.388264603422,616.110565160533,-24.0221601717603)) ;
#46662=CARTESIAN_POINT('',(193.388264603422,616.710565160533,-24.0221601717603)) ;
#46663=CARTESIAN_POINT('',(192.388264603422,616.110565160533,-25.0221601717603)) ;
#46664=CARTESIAN_POINT('Origin',(193.388264603422,616.110565160533,-25.0221601717603)) ;
#46665=CARTESIAN_POINT('',(192.388264603422,616.710565160533,-25.0221601717603)) ;
#46666=CARTESIAN_POINT('Origin',(196.738527625422,616.710565160533,-24.0221601717605)) ;
#46667=CARTESIAN_POINT('',(196.238527625422,616.110565160533,-24.0221601717605)) ;
#46668=CARTESIAN_POINT('',(196.238527625412,561.210565160533,-24.0221601717605)) ;
#46669=CARTESIAN_POINT('',(203.313527625422,616.110565160532,-24.0221601717608)) ;
#46670=CARTESIAN_POINT('Origin',(193.388264603422,616.710565160533,-25.0221601717603)) ;
#46671=CARTESIAN_POINT('',(193.388264603422,616.710565160533,-24.0221601717603)) ;
#46672=CARTESIAN_POINT('',(192.388264603422,616.710565160533,-25.0221601717603)) ;
#46673=CARTESIAN_POINT('Origin',(196.738527625422,616.710565160533,-24.0221601717605)) ;
#46674=CARTESIAN_POINT('',(196.238527625422,616.460565160533,-24.0221601717605)) ;
#46675=CARTESIAN_POINT('Origin',(0.138527625417808,588.897292039156,-20.2721601717516)) ;
#46676=CARTESIAN_POINT('',(-0.611472374596262,508.710565160568,-20.2721601717515)) ;
#46677=CARTESIAN_POINT('',(0.138527625403757,508.710565160567,-19.5221601717516)) ;
#46678=CARTESIAN_POINT('Origin',(0.138527625403723,508.710565160567,-20.2721601717516)) ;
#46679=CARTESIAN_POINT('',(0.138527625422196,613.710565160567,-19.5221601717516)) ;
#46680=CARTESIAN_POINT('',(0.138527625417842,588.897292039156,-19.5221601717516)) ;
#46681=CARTESIAN_POINT('',(-0.611472374577818,613.710565160567,-20.2721601717515)) ;
#46682=CARTESIAN_POINT('Origin',(0.138527625422167,613.710565160567,-20.2721601717516)) ;
#46683=CARTESIAN_POINT('',(-0.611472374582177,588.897292039156,-20.2721601717515)) ;
#46684=CARTESIAN_POINT('Origin',(-0.611472374578105,613.710565160567,-19.5221601717515)) ;
#46685=CARTESIAN_POINT('',(101.388527625422,613.710565160549,-19.5221601717562)) ;
#46686=CARTESIAN_POINT('',(-0.0114723745782475,613.710565160567,-23.0221601717516)) ;
#46687=CARTESIAN_POINT('',(-0.011472374579224,613.710565160567,-44.5221601717516)) ;
#46688=CARTESIAN_POINT('',(-0.611472374577943,613.710565160567,-23.0221601717515)) ;
#46689=CARTESIAN_POINT('',(99.3135276254217,613.71056516055,-23.0221601717561)) ;
#46690=CARTESIAN_POINT('',(-0.611472374578124,613.710565160567,-27.0096601717536)) ;
#46691=CARTESIAN_POINT('Origin',(205.888527625422,616.210565160531,-19.5221601717609)) ;
#46692=CARTESIAN_POINT('',(0.238527625403435,508.710565160567,-19.5221601717516)) ;
#46693=CARTESIAN_POINT('',(101.763527625403,508.71056516055,-19.5221601717562)) ;
#46694=CARTESIAN_POINT('',(0.238527625403151,506.960565160567,-19.5221601717516)) ;
#46695=CARTESIAN_POINT('',(196.838527625403,506.560565160533,-19.5221601717605)) ;
#46696=CARTESIAN_POINT('',(196.838527625403,506.560565160533,-19.5221601717605)) ;
#46697=CARTESIAN_POINT('',(196.838527625422,615.860565160533,-19.5221601717605)) ;
#46698=CARTESIAN_POINT('',(196.838527625422,615.360565160533,-19.5221601717605)) ;
#46699=CARTESIAN_POINT('',(196.738527625422,615.860565160533,-19.5221601717605)) ;
#46700=CARTESIAN_POINT('',(196.738527625422,615.860565160533,-19.5221601717605)) ;
#46701=CARTESIAN_POINT('',(196.738527625422,615.460565160533,-19.5221601717605)) ;
#46702=CARTESIAN_POINT('',(68.189609074102,544.044531662882,-19.5221601728758)) ;
#46703=CARTESIAN_POINT('',(48.6516117532406,563.582528983677,-19.5221601717538)) ;
#46704=CARTESIAN_POINT('Origin',(44.9784504245142,540.371370334153,-19.5221601717533)) ;
#46705=CARTESIAN_POINT('',(49.4331354401999,568.521073377188,-19.5221601717538)) ;
#46706=CARTESIAN_POINT('Origin',(49.0423735967098,566.051801180334,-19.5221601717518)) ;
#46707=CARTESIAN_POINT('',(73.1281535186845,544.826055026706,-19.5221601728761)) ;
#46708=CARTESIAN_POINT('Origin',(44.9784504245142,540.371370334153,-19.5221601717536)) ;
#46709=CARTESIAN_POINT('Origin',(70.6588813175403,544.435293211585,-19.5221601742775)) ;
#46710=CARTESIAN_POINT('',(17.3918523583282,565.591787903562,-19.5221601717524)) ;
#46711=CARTESIAN_POINT('Origin',(19.8918523583282,565.591787908239,-19.5221601717525)) ;
#46712=CARTESIAN_POINT('',(67.3918523583194,515.591787864358,-19.5221601717546)) ;
#46713=CARTESIAN_POINT('Origin',(69.8918523583194,515.59178790823,-19.5221601717547)) ;
#46714=CARTESIAN_POINT('',(158.588527625419,594.710565160539,-19.5221601717588)) ;
#46715=CARTESIAN_POINT('',(161.588527625419,594.710565160539,-19.5221601717589)) ;
#46716=CARTESIAN_POINT('Origin',(160.088527625419,594.710565160539,-19.5221601717588)) ;
#46717=CARTESIAN_POINT('',(161.588527625415,572.710565160539,-19.5221601717589)) ;
#46718=CARTESIAN_POINT('',(161.588527625415,572.710565160539,-19.5221601717589)) ;
#46719=CARTESIAN_POINT('',(158.588527625415,572.710565160539,-19.5221601717588)) ;
#46720=CARTESIAN_POINT('Origin',(160.088527625415,572.710565160539,-19.5221601717588)) ;
#46721=CARTESIAN_POINT('',(158.588527625419,594.710565160539,-19.5221601717588)) ;
#46722=CARTESIAN_POINT('',(165.588527625419,594.710565160538,-19.5221601717591)) ;
#46723=CARTESIAN_POINT('',(168.588527625419,594.710565160538,-19.5221601717592)) ;
#46724=CARTESIAN_POINT('Origin',(167.088527625419,594.710565160538,-19.5221601717592)) ;
#46725=CARTESIAN_POINT('',(168.588527625415,572.710565160538,-19.5221601717592)) ;
#46726=CARTESIAN_POINT('',(168.588527625415,572.710565160538,-19.5221601717592)) ;
#46727=CARTESIAN_POINT('',(165.588527625415,572.710565160538,-19.5221601717591)) ;
#46728=CARTESIAN_POINT('Origin',(167.088527625415,572.710565160538,-19.5221601717592)) ;
#46729=CARTESIAN_POINT('',(165.588527625419,594.710565160538,-19.5221601717591)) ;
#46730=CARTESIAN_POINT('',(172.588527625419,594.710565160537,-19.5221601717594)) ;
#46731=CARTESIAN_POINT('',(175.588527625419,594.710565160536,-19.5221601717595)) ;
#46732=CARTESIAN_POINT('Origin',(174.088527625419,594.710565160537,-19.5221601717595)) ;
#46733=CARTESIAN_POINT('',(175.588527625415,572.710565160536,-19.5221601717595)) ;
#46734=CARTESIAN_POINT('',(175.588527625415,572.710565160536,-19.5221601717595)) ;
#46735=CARTESIAN_POINT('',(172.588527625415,572.710565160537,-19.5221601717594)) ;
#46736=CARTESIAN_POINT('Origin',(174.088527625415,572.710565160537,-19.5221601717595)) ;
#46737=CARTESIAN_POINT('',(172.588527625419,594.710565160537,-19.5221601717594)) ;
#46738=CARTESIAN_POINT('',(158.588527625411,549.710565160539,-19.5221601717588)) ;
#46739=CARTESIAN_POINT('',(161.588527625411,549.710565160539,-19.5221601717589)) ;
#46740=CARTESIAN_POINT('Origin',(160.088527625411,549.710565160539,-19.5221601717588)) ;
#46741=CARTESIAN_POINT('',(161.588527625407,527.710565160539,-19.5221601717589)) ;
#46742=CARTESIAN_POINT('',(161.588527625407,527.710565160539,-19.5221601717589)) ;
#46743=CARTESIAN_POINT('',(158.588527625407,527.710565160539,-19.5221601717588)) ;
#46744=CARTESIAN_POINT('Origin',(160.088527625407,527.710565160539,-19.5221601717588)) ;
#46745=CARTESIAN_POINT('',(158.588527625411,549.710565160539,-19.5221601717588)) ;
#46746=CARTESIAN_POINT('',(168.588527625407,527.710565160538,-19.5221601717592)) ;
#46747=CARTESIAN_POINT('',(165.588527625407,527.710565160538,-19.5221601717591)) ;
#46748=CARTESIAN_POINT('Origin',(167.088527625407,527.710565160538,-19.5221601717592)) ;
#46749=CARTESIAN_POINT('',(165.588527625411,549.710565160538,-19.5221601717591)) ;
#46750=CARTESIAN_POINT('',(165.588527625411,549.710565160538,-19.5221601717591)) ;
#46751=CARTESIAN_POINT('',(168.588527625411,549.710565160538,-19.5221601717592)) ;
#46752=CARTESIAN_POINT('Origin',(167.088527625411,549.710565160538,-19.5221601717592)) ;
#46753=CARTESIAN_POINT('',(168.588527625407,527.710565160538,-19.5221601717592)) ;
#46754=CARTESIAN_POINT('',(172.588527625411,549.710565160537,-19.5221601717594)) ;
#46755=CARTESIAN_POINT('',(175.588527625411,549.710565160536,-19.5221601717595)) ;
#46756=CARTESIAN_POINT('Origin',(174.088527625411,549.710565160537,-19.5221601717595)) ;
#46757=CARTESIAN_POINT('',(175.588527625407,527.710565160536,-19.5221601717595)) ;
#46758=CARTESIAN_POINT('',(175.588527625407,527.710565160536,-19.5221601717595)) ;
#46759=CARTESIAN_POINT('',(172.588527625407,527.710565160537,-19.5221601717594)) ;
#46760=CARTESIAN_POINT('Origin',(174.088527625407,527.710565160537,-19.5221601717595)) ;
#46761=CARTESIAN_POINT('',(172.588527625411,549.710565160537,-19.5221601717594)) ;
#46762=CARTESIAN_POINT('',(50.0586926677957,539.082949664376,-19.5221601717538)) ;
#46763=CARTESIAN_POINT('Origin',(51.4729062301691,540.497163226748,-19.5221601717539)) ;
#46764=CARTESIAN_POINT('',(43.5642368621326,532.593195741101,-19.5221601717536)) ;
#46765=CARTESIAN_POINT('Origin',(44.9784504245059,534.007409303474,-19.5221601717536)) ;
#46766=CARTESIAN_POINT('',(37.0744829388654,539.087651546757,-19.5221601717532)) ;
#46767=CARTESIAN_POINT('Origin',(38.4886965012388,540.50186510913,-19.5221601717533)) ;
#46768=CARTESIAN_POINT('',(43.5689387445145,545.577405470032,-19.5221601717535)) ;
#46769=CARTESIAN_POINT('Origin',(44.9831523068879,546.991619032405,-19.5221601717536)) ;
#46770=CARTESIAN_POINT('',(31.8295857683906,548.578523205569,-19.522160171753)) ;
#46771=CARTESIAN_POINT('',(31.8295857683879,532.164217462742,-19.522160171753)) ;
#46772=CARTESIAN_POINT('Origin',(44.9784504245141,540.371370334153,-19.5221601717536)) ;
#46773=CARTESIAN_POINT('',(26.7397026756914,528.987255060894,-19.5221601717528)) ;
#46774=CARTESIAN_POINT('Origin',(29.2846442220396,530.575736261818,-19.5221601717601)) ;
#46775=CARTESIAN_POINT('',(26.7397026756954,551.755485607418,-19.5221601717528)) ;
#46776=CARTESIAN_POINT('Origin',(44.978450424514,540.371370334153,-19.5221601717575)) ;
#46777=CARTESIAN_POINT('Origin',(29.284644222043,550.167004406493,-19.5221601717549)) ;
#46778=CARTESIAN_POINT('',(36.7712975530987,527.22250567803,-19.5221601717532)) ;
#46779=CARTESIAN_POINT('',(33.5943351512492,522.132622585334,-19.5221601717531)) ;
#46780=CARTESIAN_POINT('Origin',(35.182816352174,524.677564131682,-19.5221601717552)) ;
#46781=CARTESIAN_POINT('',(53.1856032959254,527.222505678027,-19.522160171754)) ;
#46782=CARTESIAN_POINT('Origin',(44.9784504245142,540.371370334153,-19.5221601717536)) ;
#46783=CARTESIAN_POINT('',(56.362565697773,522.13262258533,-19.5221601717541)) ;
#46784=CARTESIAN_POINT('Origin',(54.7740844968491,524.677564131679,-19.5221601717613)) ;
#46785=CARTESIAN_POINT('Origin',(44.9784504245142,540.371370334153,-19.5221601717575)) ;
#46786=CARTESIAN_POINT('',(58.1273150806378,532.164217462738,-19.5221601717542)) ;
#46787=CARTESIAN_POINT('',(63.217198173333,528.987255060888,-19.5221601717544)) ;
#46788=CARTESIAN_POINT('Origin',(60.6722566269854,530.575736261813,-19.5221601717564)) ;
#46789=CARTESIAN_POINT('',(58.1273150806405,548.578523205564,-19.5221601717542)) ;
#46790=CARTESIAN_POINT('Origin',(44.9784504245143,540.371370334153,-19.5221601717536)) ;
#46791=CARTESIAN_POINT('',(63.217198173337,551.755485607412,-19.5221601717544)) ;
#46792=CARTESIAN_POINT('Origin',(60.6722566269888,550.167004406488,-19.5221601717615)) ;
#46793=CARTESIAN_POINT('Origin',(44.9784504245144,540.371370334153,-19.5221601717575)) ;
#46794=CARTESIAN_POINT('',(53.1856032959298,553.520234990277,-19.522160171754)) ;
#46795=CARTESIAN_POINT('',(56.3625656977793,558.610118082972,-19.5221601717541)) ;
#46796=CARTESIAN_POINT('Origin',(54.7740844968545,556.065176536624,-19.5221601717561)) ;
#46797=CARTESIAN_POINT('',(36.7712975531031,553.52023499028,-19.5221601717532)) ;
#46798=CARTESIAN_POINT('Origin',(44.9784504245142,540.371370334153,-19.5221601717536)) ;
#46799=CARTESIAN_POINT('',(33.5943351512555,558.610118082976,-19.5221601717531)) ;
#46800=CARTESIAN_POINT('Origin',(35.1828163521794,556.065176536628,-19.5221601717604)) ;
#46801=CARTESIAN_POINT('Origin',(44.9784504245142,540.371370334153,-19.5221601717575)) ;
#46802=CARTESIAN_POINT('',(41.3053508856094,563.582538762398,-19.5221601670358)) ;
#46803=CARTESIAN_POINT('',(21.7672917749906,544.04453166288,-19.5221601717525)) ;
#46804=CARTESIAN_POINT('Origin',(44.9784504245142,540.371370334153,-19.5221601717533)) ;
#46805=CARTESIAN_POINT('',(16.8287473814797,544.826055349839,-19.5221601717524)) ;
#46806=CARTESIAN_POINT('Origin',(19.2980195783332,544.435293506349,-19.5221601717457)) ;
#46807=CARTESIAN_POINT('',(40.5237715662165,568.521074351593,-19.5221601670422)) ;
#46808=CARTESIAN_POINT('Origin',(44.9784504245142,540.371370334153,-19.5221601717536)) ;
#46809=CARTESIAN_POINT('Origin',(40.9145328695602,566.05180206946,-19.5221601615182)) ;
#46810=CARTESIAN_POINT('',(21.7672748311997,536.698316068459,-19.5221601717524)) ;
#46811=CARTESIAN_POINT('',(41.3052890957879,517.16021168463,-19.5221601717534)) ;
#46812=CARTESIAN_POINT('Origin',(44.9784504245142,540.371370334153,-19.5221601717533)) ;
#46813=CARTESIAN_POINT('',(40.523765408828,512.221667291119,-19.5221601717534)) ;
#46814=CARTESIAN_POINT('Origin',(40.9145272523186,514.690939487972,-19.5221601717542)) ;
#46815=CARTESIAN_POINT('',(16.8287456930818,535.916695987675,-19.5221601717523)) ;
#46816=CARTESIAN_POINT('Origin',(44.9784504245142,540.371370334153,-19.5221601717536)) ;
#46817=CARTESIAN_POINT('Ctrl Pts',(21.7672748300875,536.698316068691,-19.5221601717526)) ;
#46818=CARTESIAN_POINT('Ctrl Pts',(21.6503315201662,537.437106614635,-19.5221601717903)) ;
#46819=CARTESIAN_POINT('Ctrl Pts',(20.7071515293286,538.794808687501,-19.5221601718653)) ;
#46820=CARTESIAN_POINT('Ctrl Pts',(18.2300981784228,538.964503729857,-19.5221601718932)) ;
#46821=CARTESIAN_POINT('Ctrl Pts',(16.8370747520978,537.437573131344,-19.522160171828)) ;
#46822=CARTESIAN_POINT('Ctrl Pts',(16.7702887385542,536.286093586995,-19.5221601717711)) ;
#46823=CARTESIAN_POINT('Ctrl Pts',(16.828745693126,535.916695987396,-19.5221601717522)) ;
#46824=CARTESIAN_POINT('',(48.6516101199294,517.160211426159,-19.5221601717537)) ;
#46825=CARTESIAN_POINT('',(68.1896090740379,536.698209005427,-19.5221601717547)) ;
#46826=CARTESIAN_POINT('Origin',(44.9784504245142,540.371370334153,-19.5221601717533)) ;
#46827=CARTESIAN_POINT('',(73.1281534675487,535.916685318467,-19.5221601717549)) ;
#46828=CARTESIAN_POINT('Origin',(70.6588812706952,536.307447161957,-19.5221601717603)) ;
#46829=CARTESIAN_POINT('',(49.4331351147273,512.221667239613,-19.5221601717538)) ;
#46830=CARTESIAN_POINT('Origin',(44.9784504245142,540.371370334153,-19.5221601717536)) ;
#46831=CARTESIAN_POINT('Ctrl Pts',(48.6516084871238,517.160211167766,-19.5221601717538)) ;
#46832=CARTESIAN_POINT('Ctrl Pts',(47.9128043995578,517.043294654392,-19.5221601721921)) ;
#46833=CARTESIAN_POINT('Ctrl Pts',(46.5550515006054,516.100143191902,-19.5221601730645)) ;
#46834=CARTESIAN_POINT('Ctrl Pts',(46.3853000863992,513.623057434898,-19.5221601733897)) ;
#46835=CARTESIAN_POINT('Ctrl Pts',(47.9122384138109,512.229997790477,-19.5221601726333)) ;
#46836=CARTESIAN_POINT('Ctrl Pts',(49.0637330000058,512.163209431194,-19.5221601719729)) ;
#46837=CARTESIAN_POINT('Ctrl Pts',(49.4331351147579,512.22166723942,-19.5221601717538)) ;
#46838=CARTESIAN_POINT('Origin',(212.38852762542,616.11056516053,-69.5221601717612)) ;
#46839=CARTESIAN_POINT('',(1.23852762542194,616.110565160567,-28.5221601717516)) ;
#46840=CARTESIAN_POINT('Origin',(1.23852762542194,616.110565160567,-27.5221601717516)) ;
#46841=CARTESIAN_POINT('',(10.4885276254219,616.110565160565,-28.5221601717516)) ;
#46842=CARTESIAN_POINT('',(106.938527625421,616.110565160549,-28.5221601717516)) ;
#46843=CARTESIAN_POINT('',(11.4885276254219,616.110565160565,-27.5221601717516)) ;
#46844=CARTESIAN_POINT('Origin',(10.4885276254219,616.110565160565,-27.5221601717516)) ;
#46845=CARTESIAN_POINT('',(11.4885276254219,616.110565160565,-25.0221601717521)) ;
#46846=CARTESIAN_POINT('',(11.4885276254219,616.110565160565,-49.0221601717564)) ;
#46847=CARTESIAN_POINT('',(12.488527625422,616.110565160565,-24.0221601717521)) ;
#46848=CARTESIAN_POINT('Origin',(12.4885276254219,616.110565160565,-25.0221601717521)) ;
#46849=CARTESIAN_POINT('',(181.388264603422,616.110565160535,-24.0221601717598)) ;
#46850=CARTESIAN_POINT('',(205.813527625422,616.110565160531,-24.0221601717609)) ;
#46851=CARTESIAN_POINT('',(182.388264603422,616.110565160535,-25.0221601717598)) ;
#46852=CARTESIAN_POINT('Origin',(181.388264603422,616.110565160536,-25.0221601717598)) ;
#46853=CARTESIAN_POINT('',(182.388264603422,616.110565160535,-27.5221601717598)) ;
#46854=CARTESIAN_POINT('',(182.388264603422,616.110565160535,-49.0221601717605)) ;
#46855=CARTESIAN_POINT('',(183.388264603422,616.110565160535,-28.5221601717598)) ;
#46856=CARTESIAN_POINT('Origin',(183.388264603422,616.110565160535,-27.5221601717598)) ;
#46857=CARTESIAN_POINT('',(191.388264603422,616.110565160534,-28.5221601717598)) ;
#46858=CARTESIAN_POINT('',(197.388396114421,616.110565160533,-28.5221601717598)) ;
#46859=CARTESIAN_POINT('',(192.388264603422,616.110565160533,-27.5221601717598)) ;
#46860=CARTESIAN_POINT('Origin',(191.388264603422,616.110565160534,-27.5221601717598)) ;
#46861=CARTESIAN_POINT('',(192.388264603422,616.110565160533,-49.1221601717605)) ;
#46862=CARTESIAN_POINT('',(196.738527625422,616.110565160533,-23.5221601717605)) ;
#46863=CARTESIAN_POINT('Origin',(196.238527625422,616.110565160533,-23.5221601717605)) ;
#46864=CARTESIAN_POINT('',(196.738527625421,616.110565160533,-44.5221601717605)) ;
#46865=CARTESIAN_POINT('',(186.138264631837,616.110565160535,-24.0200627128237)) ;
#46866=CARTESIAN_POINT('Origin',(187.388264603422,616.110565160534,-24.0203292412001)) ;
#46867=CARTESIAN_POINT('',(7.73852762542192,616.110565160566,-24.0221601717538)) ;
#46868=CARTESIAN_POINT('Origin',(6.48852762542192,616.110565160566,-24.0221601717538)) ;
#46869=CARTESIAN_POINT('Origin',(-0.0114723745895816,561.210565160567,-69.5221601717516)) ;
#46870=CARTESIAN_POINT('',(-0.0114723745966916,508.710565160567,-23.0221601717516)) ;
#46871=CARTESIAN_POINT('',(-0.0114723745976681,508.710565160567,-44.5221601717516)) ;
#46872=CARTESIAN_POINT('',(-0.0114723745966299,509.210565160567,-23.5221601717516)) ;
#46873=CARTESIAN_POINT('Origin',(-0.0114723745966039,509.210565160567,-23.0221601717516)) ;
#46874=CARTESIAN_POINT('',(-0.0114723745783614,613.210565160567,-23.5221601717515)) ;
#46875=CARTESIAN_POINT('',(-0.0114723745923263,533.710565160567,-23.5221601717516)) ;
#46876=CARTESIAN_POINT('Origin',(-0.0114723745783429,613.210565160567,-23.0221601717516)) ;
#46877=CARTESIAN_POINT('Origin',(49.042373596694,566.051801180341,-256.918732177553)) ;
#46878=CARTESIAN_POINT('',(49.4331354401894,568.521073377188,-256.918732177553)) ;
#46879=CARTESIAN_POINT('',(48.6516117532405,563.582528983677,-20.2721601717532)) ;
#46880=CARTESIAN_POINT('Origin',(44.9784504245142,540.371370334153,-19.5221601717536)) ;
#46881=CARTESIAN_POINT('',(73.1281535186845,544.826055026706,-19.5221601717548)) ;
#46882=CARTESIAN_POINT('Origin',(40.9145328695602,566.05180206946,-19.5221601717534)) ;
#46883=CARTESIAN_POINT('',(40.5237715662164,568.521074351593,-19.5221601717534)) ;
#46884=CARTESIAN_POINT('',(41.3053508855747,563.582538762618,-19.5221601717534)) ;
#46885=CARTESIAN_POINT('Origin',(44.9784504245142,540.371370334153,-19.5221601717536)) ;
#46886=CARTESIAN_POINT('',(16.8287473814692,544.826055349839,-256.918732177552)) ;
#46887=CARTESIAN_POINT('Origin',(19.2980195783158,544.435293506344,-256.918732177552)) ;
#46888=CARTESIAN_POINT('',(21.7672917749906,544.04453166288,-20.272160171752)) ;
#46889=CARTESIAN_POINT('Ctrl Pts',(21.7672748300875,536.698316068691,-19.5221601716228)) ;
#46890=CARTESIAN_POINT('Ctrl Pts',(21.7672748301048,536.698316068582,-19.7221601716661)) ;
#46891=CARTESIAN_POINT('Ctrl Pts',(21.7672748296538,536.698316071431,-19.9221601717093)) ;
#46892=CARTESIAN_POINT('Ctrl Pts',(21.7672748296711,536.698316071321,-20.1221601717526)) ;
#46893=CARTESIAN_POINT('Ctrl Pts',(21.6503315201662,537.437106614635,-19.5221601716605)) ;
#46894=CARTESIAN_POINT('Ctrl Pts',(21.6503315202122,537.43710661454,-19.7221601717038)) ;
#46895=CARTESIAN_POINT('Ctrl Pts',(21.6503315190249,537.437106617018,-19.922160171747)) ;
#46896=CARTESIAN_POINT('Ctrl Pts',(21.6503315190709,537.437106616922,-20.1221601717903)) ;
#46897=CARTESIAN_POINT('Ctrl Pts',(20.7071515293285,538.794808687501,-19.5221601717356)) ;
#46898=CARTESIAN_POINT('Ctrl Pts',(20.7071515294062,538.794808687459,-19.7221601717788)) ;
#46899=CARTESIAN_POINT('Ctrl Pts',(20.7071515273852,538.794808688543,-19.9221601718221)) ;
#46900=CARTESIAN_POINT('Ctrl Pts',(20.707151527463,538.794808688501,-20.1221601718653)) ;
#46901=CARTESIAN_POINT('Ctrl Pts',(18.2300981784228,538.964503729856,-19.5221601717634)) ;
#46902=CARTESIAN_POINT('Ctrl Pts',(18.230098178466,538.964503729874,-19.7221601718066)) ;
#46903=CARTESIAN_POINT('Ctrl Pts',(18.2300981773464,538.964503729414,-19.9221601718499)) ;
#46904=CARTESIAN_POINT('Ctrl Pts',(18.2300981773896,538.964503729431,-20.1221601718932)) ;
#46905=CARTESIAN_POINT('Ctrl Pts',(16.8370747520978,537.437573131345,-19.5221601716982)) ;
#46906=CARTESIAN_POINT('Ctrl Pts',(16.8370747521019,537.437573131355,-19.7221601717414)) ;
#46907=CARTESIAN_POINT('Ctrl Pts',(16.8370747519932,537.437573131106,-19.9221601717847)) ;
#46908=CARTESIAN_POINT('Ctrl Pts',(16.8370747519973,537.437573131115,-20.122160171828)) ;
#46909=CARTESIAN_POINT('Ctrl Pts',(16.7702887385542,536.286093586995,-19.5221601716413)) ;
#46910=CARTESIAN_POINT('Ctrl Pts',(16.7702887385554,536.286093586989,-19.7221601716846)) ;
#46911=CARTESIAN_POINT('Ctrl Pts',(16.7702887385333,536.286093587149,-19.9221601717279)) ;
#46912=CARTESIAN_POINT('Ctrl Pts',(16.7702887385344,536.286093587143,-20.1221601717712)) ;
#46913=CARTESIAN_POINT('Ctrl Pts',(16.828745693126,535.916695987396,-19.5221601716224)) ;
#46914=CARTESIAN_POINT('Ctrl Pts',(16.8287456931277,535.916695987385,-19.7221601716657)) ;
#46915=CARTESIAN_POINT('Ctrl Pts',(16.8287456930828,535.916695987669,-19.922160171709)) ;
#46916=CARTESIAN_POINT('Ctrl Pts',(16.8287456930845,535.916695987658,-20.1221601717523)) ;
#46917=CARTESIAN_POINT('',(16.828745693126,535.916695987396,-19.5221601716224)) ;
#46918=CARTESIAN_POINT('',(21.7672748296711,536.698316071321,-20.1221601717508)) ;
#46919=CARTESIAN_POINT('Origin',(44.9784504245142,540.371370334153,-19.5221601717536)) ;
#46920=CARTESIAN_POINT('',(40.5237654088175,512.221667291119,-256.918732177553)) ;
#46921=CARTESIAN_POINT('Origin',(40.9145272523129,514.690939487966,-256.918732177553)) ;
#46922=CARTESIAN_POINT('',(41.3052890957878,517.16021168463,-20.2721601717529)) ;
#46923=CARTESIAN_POINT('Ctrl Pts',(48.6516084871238,517.160211167766,-19.5221601702455)) ;
#46924=CARTESIAN_POINT('Ctrl Pts',(48.6516084883974,517.160211167967,-19.7221601707483)) ;
#46925=CARTESIAN_POINT('Ctrl Pts',(48.651608489671,517.160211168169,-19.922160171251)) ;
#46926=CARTESIAN_POINT('Ctrl Pts',(48.6516084909445,517.16021116837,-20.1221601717538)) ;
#46927=CARTESIAN_POINT('Ctrl Pts',(47.9128043995578,517.043294654392,-19.5221601706839)) ;
#46928=CARTESIAN_POINT('Ctrl Pts',(47.9128044006695,517.043294654927,-19.7221601711867)) ;
#46929=CARTESIAN_POINT('Ctrl Pts',(47.9128044017683,517.043294655448,-19.9221601716894)) ;
#46930=CARTESIAN_POINT('Ctrl Pts',(47.91280440288,517.043294655983,-20.1221601721921)) ;
#46931=CARTESIAN_POINT('Ctrl Pts',(46.5550515006053,516.100143191901,-19.5221601715563)) ;
#46932=CARTESIAN_POINT('Ctrl Pts',(46.555051501089,516.100143192805,-19.722160172059)) ;
#46933=CARTESIAN_POINT('Ctrl Pts',(46.5550515015749,516.100143193707,-19.9221601725618)) ;
#46934=CARTESIAN_POINT('Ctrl Pts',(46.5550515020586,516.100143194611,-20.1221601730645)) ;
#46935=CARTESIAN_POINT('Ctrl Pts',(46.3853000863992,513.623057434898,-19.5221601718814)) ;
#46936=CARTESIAN_POINT('Ctrl Pts',(46.3853000861961,513.623057435401,-19.7221601723842)) ;
#46937=CARTESIAN_POINT('Ctrl Pts',(46.385300085985,513.623057435896,-19.922160172887)) ;
#46938=CARTESIAN_POINT('Ctrl Pts',(46.385300085782,513.623057436399,-20.1221601733897)) ;
#46939=CARTESIAN_POINT('Ctrl Pts',(47.912238413811,512.229997790477,-19.5221601711252)) ;
#46940=CARTESIAN_POINT('Ctrl Pts',(47.9122384136994,512.229997790525,-19.7221601716279)) ;
#46941=CARTESIAN_POINT('Ctrl Pts',(47.9122384135884,512.229997790576,-19.9221601721307)) ;
#46942=CARTESIAN_POINT('Ctrl Pts',(47.9122384134769,512.229997790623,-20.1221601726335)) ;
#46943=CARTESIAN_POINT('Ctrl Pts',(49.0637330000058,512.163209431194,-19.5221601704647)) ;
#46944=CARTESIAN_POINT('Ctrl Pts',(49.0637330000785,512.163209431207,-19.7221601709675)) ;
#46945=CARTESIAN_POINT('Ctrl Pts',(49.0637330001476,512.163209431209,-19.9221601714703)) ;
#46946=CARTESIAN_POINT('Ctrl Pts',(49.0637330002203,512.163209431222,-20.122160171973)) ;
#46947=CARTESIAN_POINT('Ctrl Pts',(49.4331351147579,512.22166723942,-19.5221601702455)) ;
#46948=CARTESIAN_POINT('Ctrl Pts',(49.4331351148848,512.22166723944,-19.7221601707483)) ;
#46949=CARTESIAN_POINT('Ctrl Pts',(49.4331351150117,512.22166723946,-19.9221601712511)) ;
#46950=CARTESIAN_POINT('Ctrl Pts',(49.4331351151386,512.22166723948,-20.1221601717539)) ;
#46951=CARTESIAN_POINT('',(49.4331351147579,512.22166723942,-19.5221601717538)) ;
#46952=CARTESIAN_POINT('',(48.6516117532324,517.160211684628,-20.2721601717537)) ;
#46953=CARTESIAN_POINT('Origin',(44.9784504245142,540.371370334153,-19.5221601717536)) ;
#46954=CARTESIAN_POINT('',(73.1281534675381,535.916685318467,-256.918732177554)) ;
#46955=CARTESIAN_POINT('Origin',(70.658881270691,536.307447161963,-256.918732177554)) ;
#46956=CARTESIAN_POINT('',(68.1896090740378,536.698209005427,-20.2721601717541)) ;
#46957=CARTESIAN_POINT('Origin',(70.6588813175403,544.435293211585,-19.5221601717547)) ;
#46958=CARTESIAN_POINT('',(68.189609074039,544.044531662871,-20.2721601717546)) ;
#46959=CARTESIAN_POINT('Origin',(99.3135276254216,613.21056516055,-23.0221601717561)) ;
#46960=CARTESIAN_POINT('',(-0.611472374578058,613.210565160567,-23.5221601717515)) ;
#46961=CARTESIAN_POINT('',(99.3135276254216,613.21056516055,-23.5221601717561)) ;
#46962=CARTESIAN_POINT('Origin',(-0.611472374578028,613.210565160567,-23.0221601717515)) ;
#46963=CARTESIAN_POINT('Origin',(199.238527625403,506.210565160532,-23.5221601717606)) ;
#46964=CARTESIAN_POINT('',(-0.611472374596327,509.210565160567,-23.5221601717515)) ;
#46965=CARTESIAN_POINT('',(99.6885276254034,509.21056516055,-23.5221601717561)) ;
#46966=CARTESIAN_POINT('',(-0.61147237459199,533.897292039156,-23.5221601717515)) ;
#46967=CARTESIAN_POINT('Origin',(99.6885276254034,509.21056516055,-23.0221601717561)) ;
#46968=CARTESIAN_POINT('',(-0.611472374596387,508.710565160568,-23.0221601717515)) ;
#46969=CARTESIAN_POINT('',(99.6885276254033,508.71056516055,-23.0221601717561)) ;
#46970=CARTESIAN_POINT('Origin',(-0.611472374596307,509.210565160567,-23.0221601717515)) ;
#46971=CARTESIAN_POINT('Origin',(0.138527625403477,508.710565160567,-19.5221601717516)) ;
#46972=CARTESIAN_POINT('',(-0.611472374596568,508.710565160568,-27.0096601717537)) ;
#46973=CARTESIAN_POINT('',(0.238527625403442,508.710565160567,-19.5221601717516)) ;
#46974=CARTESIAN_POINT('Origin',(196.238527625422,616.460565160533,-23.5221601717605)) ;
#46975=CARTESIAN_POINT('Origin',(204.238527625403,507.060565160531,-25.4221601717608)) ;
#46976=CARTESIAN_POINT('',(196.988527625403,506.560565160533,-25.4221601717605)) ;
#46977=CARTESIAN_POINT('',(196.988527625403,507.060565160533,-25.9221601717605)) ;
#46978=CARTESIAN_POINT('Origin',(196.988527625403,507.060565160533,-25.4221601717605)) ;
#46979=CARTESIAN_POINT('',(197.588527625403,507.060565160533,-25.9221601717605)) ;
#46980=CARTESIAN_POINT('',(204.238527625403,507.060565160531,-25.9221601717608)) ;
#46981=CARTESIAN_POINT('',(197.588527625403,506.560565160533,-25.4221601717605)) ;
#46982=CARTESIAN_POINT('Origin',(197.588527625403,507.060565160533,-25.4221601717605)) ;
#46983=CARTESIAN_POINT('',(204.238527625403,506.560565160532,-25.4221601717608)) ;
#46984=CARTESIAN_POINT('Origin',(208.388527625422,616.210565160531,-25.922160171761)) ;
#46985=CARTESIAN_POINT('',(196.988527625422,615.360565160533,-25.9221601717605)) ;
#46986=CARTESIAN_POINT('',(196.988527625422,616.210565160533,-25.9221601717605)) ;
#46987=CARTESIAN_POINT('',(197.588527625422,615.360565160533,-25.9221601717605)) ;
#46988=CARTESIAN_POINT('',(203.863527625422,615.360565160531,-25.9221601717608)) ;
#46989=CARTESIAN_POINT('',(197.588527625422,616.068993308983,-25.9221601717605)) ;
#46990=CARTESIAN_POINT('Origin',(196.988527625421,616.210565160533,-43.5221601717605)) ;
#46991=CARTESIAN_POINT('',(196.988527625403,506.560565160533,-20.3721601717605)) ;
#46992=CARTESIAN_POINT('',(196.988527625403,506.560565160533,-31.5221601717605)) ;
#46993=CARTESIAN_POINT('',(196.988527625422,615.860565160533,-20.3721601717605)) ;
#46994=CARTESIAN_POINT('',(196.988527625422,616.210565160533,-20.3721601717605)) ;
#46995=CARTESIAN_POINT('',(196.988527625422,615.860565160533,-25.4221601717605)) ;
#46996=CARTESIAN_POINT('',(196.988527625422,615.860565160533,-31.5221601717605)) ;
#46997=CARTESIAN_POINT('Origin',(196.988527625422,615.360565160533,-25.4221601717605)) ;
#46998=CARTESIAN_POINT('Origin',(203.863527625422,615.360565160531,-25.4221601717608)) ;
#46999=CARTESIAN_POINT('',(197.588527625422,615.860565160533,-25.4221601717605)) ;
#47000=CARTESIAN_POINT('Origin',(197.588527625422,615.360565160533,-25.4221601717605)) ;
#47001=CARTESIAN_POINT('',(203.863527625422,615.860565160531,-25.4221601717608)) ;
#47002=CARTESIAN_POINT('Origin',(199.338527625422,615.860565160532,-19.5221601717606)) ;
#47003=CARTESIAN_POINT('',(197.588527625422,615.860565160533,-20.2721601717605)) ;
#47004=CARTESIAN_POINT('Origin',(196.838527625422,615.860565160533,-20.2721601717605)) ;
#47005=CARTESIAN_POINT('',(197.588527625422,615.860565160533,-20.2721601717605)) ;
#47006=CARTESIAN_POINT('Origin',(196.738527625422,615.860565160533,-20.3721601717605)) ;
#47007=CARTESIAN_POINT('',(196.738527625422,615.860565160533,-19.5221601717605)) ;
#47008=CARTESIAN_POINT('Origin',(196.238527625412,561.210565160533,-23.5221601717605)) ;
#47009=CARTESIAN_POINT('',(196.738527625412,561.210565160533,-23.5221601717605)) ;
#47010=CARTESIAN_POINT('Origin',(196.738527625422,616.210565160533,-19.5221601717605)) ;
#47011=CARTESIAN_POINT('Origin',(191.388264603412,561.460565160534,-27.5221601717602)) ;
#47012=CARTESIAN_POINT('',(191.388264603412,561.460565160534,-28.5221601717602)) ;
#47013=CARTESIAN_POINT('',(192.388264603412,561.460565160534,-27.5221601717602)) ;
#47014=CARTESIAN_POINT('Origin',(199.238527625403,506.210565160532,-28.5221601717606)) ;
#47015=CARTESIAN_POINT('',(183.388264603403,506.335565160535,-28.5221601717599)) ;
#47016=CARTESIAN_POINT('Origin',(181.388264603403,506.460565160535,-25.0221601717598)) ;
#47017=CARTESIAN_POINT('',(182.388264603403,506.460565160535,-25.0221601717598)) ;
#47018=CARTESIAN_POINT('',(181.388264603403,506.460565160535,-24.0221601717598)) ;
#47019=CARTESIAN_POINT('Origin',(182.388264603403,506.460565160535,-28.5221601717599)) ;
#47020=CARTESIAN_POINT('',(182.388264603403,506.335565160535,-27.5221601717599)) ;
#47021=CARTESIAN_POINT('Origin',(183.388264603403,506.335565160535,-27.5221601717599)) ;
#47022=CARTESIAN_POINT('Origin',(10.4885276254026,506.335565160565,-27.522160171752)) ;
#47023=CARTESIAN_POINT('',(10.4885276254026,506.335565160565,-28.522160171752)) ;
#47024=CARTESIAN_POINT('',(11.4885276254026,506.335565160565,-27.522160171752)) ;
#47025=CARTESIAN_POINT('Origin',(199.238527625403,506.210565160532,-28.5221601717606)) ;
#47026=CARTESIAN_POINT('',(1.2385276254122,560.835565160567,-28.5221601717516)) ;
#47027=CARTESIAN_POINT('Origin',(12.4885276254027,506.460565160565,-25.0221601717521)) ;
#47028=CARTESIAN_POINT('',(12.4885276254027,506.460565160565,-24.0221601717521)) ;
#47029=CARTESIAN_POINT('',(11.4885276254027,506.460565160565,-25.0221601717521)) ;
#47030=CARTESIAN_POINT('Origin',(182.388264603403,506.460565160535,-24.0221601717598)) ;
#47031=CARTESIAN_POINT('Origin',(1.23852762541224,560.835565160567,-27.5221601717516)) ;
#47032=CARTESIAN_POINT('',(0.238527625412235,560.835565160567,-27.5221601717516)) ;
#47033=CARTESIAN_POINT('Origin',(12.4885276254123,561.460565160565,-25.0221601717521)) ;
#47034=CARTESIAN_POINT('',(11.4885276254123,561.460565160565,-25.0221601717521)) ;
#47035=CARTESIAN_POINT('',(12.4885276254124,561.460565160565,-24.0221601717521)) ;
#47036=CARTESIAN_POINT('Origin',(11.488527625422,616.710565160565,-28.5221601717516)) ;
#47037=CARTESIAN_POINT('',(11.488527625422,616.710565160565,-27.5221601717516)) ;
#47038=CARTESIAN_POINT('Origin',(10.488527625422,616.710565160565,-27.5221601717516)) ;
#47039=CARTESIAN_POINT('',(10.488527625422,616.710565160565,-28.5221601717516)) ;
#47040=CARTESIAN_POINT('Origin',(1.48852762542202,616.710565160567,-28.5221601717516)) ;
#47041=CARTESIAN_POINT('',(1.23852762542194,616.085565160567,-28.5221601717516)) ;
#47042=CARTESIAN_POINT('Origin',(1.23852762542194,616.085565160567,-27.5221601717516)) ;
#47043=CARTESIAN_POINT('Origin',(181.388264603412,561.460565160536,-25.0221601717598)) ;
#47044=CARTESIAN_POINT('',(182.388264603412,561.460565160535,-25.0221601717598)) ;
#47045=CARTESIAN_POINT('',(181.388264603412,561.460565160536,-24.0221601717598)) ;
#47046=CARTESIAN_POINT('Origin',(182.388264603422,616.710565160535,-28.5221601717598)) ;
#47047=CARTESIAN_POINT('',(182.388264603422,616.710565160535,-27.5221601717598)) ;
#47048=CARTESIAN_POINT('Origin',(183.388264603422,616.710565160535,-27.5221601717598)) ;
#47049=CARTESIAN_POINT('',(183.388264603422,616.710565160535,-28.5221601717598)) ;
#47050=CARTESIAN_POINT('Origin',(192.388264603422,616.710565160533,-24.0221601717603)) ;
#47051=CARTESIAN_POINT('',(192.388264603422,616.710565160533,-27.5221601717598)) ;
#47052=CARTESIAN_POINT('Origin',(191.388264603422,616.710565160534,-27.5221601717598)) ;
#47053=CARTESIAN_POINT('',(191.388264603422,616.710565160534,-28.5221601717598)) ;
#47054=CARTESIAN_POINT('Origin',(182.388264603422,616.710565160535,-28.5221601717598)) ;
#47055=CARTESIAN_POINT('Origin',(196.738527625422,616.210565160533,-20.3721601717605)) ;
#47056=CARTESIAN_POINT('Origin',(196.738527625403,506.560565160533,-20.3721601717605)) ;
#47057=CARTESIAN_POINT('Origin',(200.088527625403,506.560565160532,-19.5221601717607)) ;
#47058=CARTESIAN_POINT('',(197.588527625403,506.560565160533,-20.2721601717605)) ;
#47059=CARTESIAN_POINT('',(197.588527625403,506.560565160533,-20.2721601717605)) ;
#47060=CARTESIAN_POINT('Origin',(196.838527625403,506.560565160533,-20.2721601717605)) ;
#47061=CARTESIAN_POINT('Origin',(0.238527625422194,615.460565160567,-19.5221601717516)) ;
#47062=CARTESIAN_POINT('Origin',(192.388264603422,616.710565160533,-24.0221601717603)) ;
#47063=CARTESIAN_POINT('Origin',(6.48852762542202,616.710565160566,-24.0221601717538)) ;
#47064=CARTESIAN_POINT('',(7.73852762542202,616.710565160566,-24.0221601717538)) ;
#47065=CARTESIAN_POINT('Origin',(187.388264603422,616.710565160534,-24.0203292412001)) ;
#47066=CARTESIAN_POINT('',(188.638264603422,616.710565160534,-24.0203292412001)) ;
#47067=CARTESIAN_POINT('Origin',(11.4885276254027,506.460565160565,-24.0221601717521)) ;
#47068=CARTESIAN_POINT('Origin',(6.48852762542202,616.710565160566,-24.0221601717538)) ;
#47069=CARTESIAN_POINT('',(7.73852762542202,616.710565160566,-24.0221601717538)) ;
#47070=CARTESIAN_POINT('Origin',(29.2846442220398,550.16700440648,-256.918732177554)) ;
#47071=CARTESIAN_POINT('',(31.8295857683906,548.578523205569,-19.5221601717539)) ;
#47072=CARTESIAN_POINT('',(26.7397026756954,551.755485607418,-19.522160171754)) ;
#47073=CARTESIAN_POINT('Origin',(29.2846442220421,530.575736261811,-256.918732177554)) ;
#47074=CARTESIAN_POINT('',(26.7397026756914,528.987255060894,-19.5221601717534)) ;
#47075=CARTESIAN_POINT('',(31.8295857683878,532.164217462742,-20.2721601717535)) ;
#47076=CARTESIAN_POINT('Origin',(44.978450424514,540.371370334142,-256.918732177554)) ;
#47077=CARTESIAN_POINT('Origin',(44.978450424514,540.371370334142,-256.918732177554)) ;
#47078=CARTESIAN_POINT('Origin',(44.9784504245044,540.371370334145,-256.918732177554)) ;
#47079=CARTESIAN_POINT('Origin',(19.8918523583282,565.591787908239,-19.6319951288125)) ;
#47080=CARTESIAN_POINT('',(17.5016873153832,565.591787908239,-19.6319951288124)) ;
#47081=CARTESIAN_POINT('Origin',(69.8918523583194,515.59178790823,-19.6319951288147)) ;
#47082=CARTESIAN_POINT('',(67.5016873153744,515.59178790823,-19.6319951288146)) ;
#47083=CARTESIAN_POINT('Origin',(199.238527625403,506.210565160532,-24.0221601717606)) ;
#47084=CARTESIAN_POINT('Origin',(-0.61147237458762,561.584018917744,-34.4971601717558)) ;
#47085=CARTESIAN_POINT('Origin',(44.983152306877,546.991619032405,-256.918732177554)) ;
#47086=CARTESIAN_POINT('',(43.5689387445037,545.577405470032,-256.918732177554)) ;
#47087=CARTESIAN_POINT('Origin',(38.4886965012279,540.50186510913,-256.918732177553)) ;
#47088=CARTESIAN_POINT('',(37.0744829388546,539.087651546757,-256.918732177553)) ;
#47089=CARTESIAN_POINT('Origin',(44.9784504244951,534.007409303474,-256.918732177554)) ;
#47090=CARTESIAN_POINT('',(43.5642368621218,532.593195741101,-256.918732177554)) ;
#47091=CARTESIAN_POINT('Origin',(51.4729062301583,540.497163226748,-256.918732177554)) ;
#47092=CARTESIAN_POINT('',(50.058692667785,539.082949664375,-256.918732177554)) ;
#47093=CARTESIAN_POINT('Origin',(174.088527625396,527.710565160537,-256.918732177559)) ;
#47094=CARTESIAN_POINT('',(175.588527625407,527.710565160536,-19.5221601717595)) ;
#47095=CARTESIAN_POINT('',(172.588527625407,527.710565160537,-20.2721601717594)) ;
#47096=CARTESIAN_POINT('Origin',(175.588527625396,527.710565160536,-256.91873217756)) ;
#47097=CARTESIAN_POINT('',(175.588527625411,549.710565160536,-20.2721601717595)) ;
#47098=CARTESIAN_POINT('Origin',(174.0885276254,549.710565160537,-256.918732177559)) ;
#47099=CARTESIAN_POINT('',(172.588527625411,549.710565160537,-19.5221601717594)) ;
#47100=CARTESIAN_POINT('Origin',(172.5885276254,549.710565160537,-256.918732177559)) ;
#47101=CARTESIAN_POINT('Origin',(167.0885276254,549.710565160538,-256.918732177559)) ;
#47102=CARTESIAN_POINT('',(165.588527625411,549.710565160538,-19.5221601717591)) ;
#47103=CARTESIAN_POINT('',(168.588527625411,549.710565160538,-20.2721601717592)) ;
#47104=CARTESIAN_POINT('Origin',(165.5885276254,549.710565160538,-256.918732177559)) ;
#47105=CARTESIAN_POINT('',(165.588527625407,527.710565160538,-20.2721601717591)) ;
#47106=CARTESIAN_POINT('Origin',(167.088527625396,527.710565160538,-256.918732177559)) ;
#47107=CARTESIAN_POINT('',(168.588527625407,527.710565160538,-19.5221601717592)) ;
#47108=CARTESIAN_POINT('Origin',(168.588527625396,527.710565160538,-256.918732177559)) ;
#47109=CARTESIAN_POINT('Origin',(160.088527625396,527.710565160539,-256.918732177559)) ;
#47110=CARTESIAN_POINT('',(161.588527625407,527.710565160539,-19.5221601717589)) ;
#47111=CARTESIAN_POINT('',(158.588527625407,527.710565160539,-20.2721601717588)) ;
#47112=CARTESIAN_POINT('Origin',(161.588527625396,527.710565160539,-256.918732177559)) ;
#47113=CARTESIAN_POINT('',(161.588527625411,549.710565160539,-20.2721601717589)) ;
#47114=CARTESIAN_POINT('Origin',(160.0885276254,549.710565160539,-256.918732177559)) ;
#47115=CARTESIAN_POINT('',(158.588527625411,549.710565160539,-19.5221601717588)) ;
#47116=CARTESIAN_POINT('Origin',(158.5885276254,549.71056516054,-256.918732177559)) ;
#47117=CARTESIAN_POINT('Origin',(174.088527625404,572.710565160537,-256.918732177559)) ;
#47118=CARTESIAN_POINT('',(175.588527625415,572.710565160536,-19.5221601717595)) ;
#47119=CARTESIAN_POINT('',(172.588527625415,572.710565160537,-20.2721601717594)) ;
#47120=CARTESIAN_POINT('Origin',(175.588527625404,572.710565160536,-256.91873217756)) ;
#47121=CARTESIAN_POINT('',(175.588527625419,594.710565160536,-20.2721601717595)) ;
#47122=CARTESIAN_POINT('Origin',(174.088527625408,594.710565160537,-256.918732177559)) ;
#47123=CARTESIAN_POINT('',(172.588527625419,594.710565160537,-19.5221601717594)) ;
#47124=CARTESIAN_POINT('Origin',(172.588527625408,594.710565160537,-256.918732177559)) ;
#47125=CARTESIAN_POINT('Origin',(167.088527625404,572.710565160538,-256.918732177559)) ;
#47126=CARTESIAN_POINT('',(168.588527625415,572.710565160538,-19.5221601717592)) ;
#47127=CARTESIAN_POINT('',(165.588527625415,572.710565160538,-20.2721601717591)) ;
#47128=CARTESIAN_POINT('Origin',(168.588527625404,572.710565160538,-256.918732177559)) ;
#47129=CARTESIAN_POINT('',(168.588527625419,594.710565160538,-20.2721601717592)) ;
#47130=CARTESIAN_POINT('Origin',(167.088527625408,594.710565160538,-256.918732177559)) ;
#47131=CARTESIAN_POINT('',(165.588527625419,594.710565160538,-19.5221601717591)) ;
#47132=CARTESIAN_POINT('Origin',(165.588527625408,594.710565160538,-256.918732177559)) ;
#47133=CARTESIAN_POINT('Origin',(160.088527625404,572.710565160539,-256.918732177559)) ;
#47134=CARTESIAN_POINT('',(161.588527625415,572.710565160539,-19.5221601717589)) ;
#47135=CARTESIAN_POINT('',(158.588527625415,572.710565160539,-20.2721601717588)) ;
#47136=CARTESIAN_POINT('Origin',(161.588527625404,572.710565160539,-256.918732177559)) ;
#47137=CARTESIAN_POINT('',(161.588527625419,594.710565160539,-20.2721601717589)) ;
#47138=CARTESIAN_POINT('Origin',(160.088527625408,594.710565160539,-256.918732177559)) ;
#47139=CARTESIAN_POINT('',(158.588527625419,594.710565160539,-19.5221601717588)) ;
#47140=CARTESIAN_POINT('Origin',(158.588527625408,594.71056516054,-256.918732177559)) ;
#47141=CARTESIAN_POINT('Origin',(196.838527625447,759.606565160533,-20.2721601717605)) ;
#47142=CARTESIAN_POINT('',(197.588527625403,507.060565160533,-20.2721601717605)) ;
#47143=CARTESIAN_POINT('Origin',(197.588527625422,615.927421457433,-27.7686821023705)) ;
#47144=CARTESIAN_POINT('Origin',(187.388264603402,504.210565160534,-24.0203292412001)) ;
#47145=CARTESIAN_POINT('',(186.138264631817,504.210565160534,-24.0200627128238)) ;
#47146=CARTESIAN_POINT('Origin',(44.9784504245116,540.371370334154,-256.918732177554)) ;
#47147=CARTESIAN_POINT('Origin',(44.9784504245024,540.371370334161,-256.918732177554)) ;
#47148=CARTESIAN_POINT('Origin',(44.9784504244953,540.371370334152,-256.918732177554)) ;
#47149=CARTESIAN_POINT('Origin',(35.1828163521764,524.67756413169,-256.918732177554)) ;
#47150=CARTESIAN_POINT('',(36.7712975530987,527.22250567803,-19.5221601717541)) ;
#47151=CARTESIAN_POINT('',(33.5943351512492,522.132622585334,-19.5221601717543)) ;
#47152=CARTESIAN_POINT('Origin',(54.774084496846,524.677564131692,-256.918732177555)) ;
#47153=CARTESIAN_POINT('',(56.362565697773,522.13262258533,-19.5221601717548)) ;
#47154=CARTESIAN_POINT('',(53.1856032959251,527.222505678027,-20.2721601717544)) ;
#47155=CARTESIAN_POINT('Origin',(44.9784504245142,540.371370334164,-256.918732177554)) ;
#47156=CARTESIAN_POINT('Origin',(44.9784504245142,540.371370334164,-256.918732177554)) ;
#47157=CARTESIAN_POINT('Origin',(60.672256626967,530.575736261826,-256.918732177555)) ;
#47158=CARTESIAN_POINT('',(58.1273150806378,532.164217462738,-19.5221601717551)) ;
#47159=CARTESIAN_POINT('',(63.217198173333,528.987255060888,-19.5221601717556)) ;
#47160=CARTESIAN_POINT('Origin',(60.6722566269648,550.167004406496,-256.918732177555)) ;
#47161=CARTESIAN_POINT('',(63.217198173337,551.755485607412,-19.5221601717551)) ;
#47162=CARTESIAN_POINT('',(58.1273150806405,548.578523205564,-20.2721601717547)) ;
#47163=CARTESIAN_POINT('Origin',(44.9784504244929,540.371370334164,-256.918732177554)) ;
#47164=CARTESIAN_POINT('Origin',(44.9784504244929,540.371370334164,-256.918732177554)) ;
#47165=CARTESIAN_POINT('Origin',(54.7740844968305,556.065176536617,-256.918732177555)) ;
#47166=CARTESIAN_POINT('',(53.1856032959298,553.520234990277,-19.5221601717548)) ;
#47167=CARTESIAN_POINT('',(56.3625656977793,558.610118082972,-19.5221601717553)) ;
#47168=CARTESIAN_POINT('Origin',(35.1828163521609,556.065176536615,-256.918732177554)) ;
#47169=CARTESIAN_POINT('',(33.5943351512555,558.610118082976,-19.5221601717537)) ;
#47170=CARTESIAN_POINT('',(36.7712975531033,553.52023499028,-20.2721601717537)) ;
#47171=CARTESIAN_POINT('Origin',(44.9784504244926,540.371370334143,-256.918732177554)) ;
#47172=CARTESIAN_POINT('Origin',(44.9784504244926,540.371370334143,-256.918732177554)) ;
#86281=UNCERTAINTY_MEASURE_WITH_UNIT(LENGTH_MEASURE(0.01),#86331,
'DISTANCE_ACCURACY_VALUE',
'Maximum model space distance between geometric entities at asserted c
onnectivities') ;
#86304=UNCERTAINTY_MEASURE_WITH_UNIT(LENGTH_MEASURE(0.01),#86331,
'DISTANCE_ACCURACY_VALUE',
'Maximum model space distance between geometric entities at asserted c
onnectivities') ;
#86307=(
GEOMETRIC_REPRESENTATION_CONTEXT(3)
GLOBAL_UNCERTAINTY_ASSIGNED_CONTEXT((#86281))
GLOBAL_UNIT_ASSIGNED_CONTEXT((#86331,#86333,#86334))
REPRESENTATION_CONTEXT('','3D')
) ;
#86330=(
GEOMETRIC_REPRESENTATION_CONTEXT(3)
GLOBAL_UNCERTAINTY_ASSIGNED_CONTEXT((#86304))
GLOBAL_UNIT_ASSIGNED_CONTEXT((#86331,#86333,#86334))
REPRESENTATION_CONTEXT('','3D')
) ;
#86331=(
LENGTH_UNIT()
NAMED_UNIT(*)
SI_UNIT(.MILLI.,.METRE.)
) ;
#86333=(
NAMED_UNIT(*)
PLANE_ANGLE_UNIT()
SI_UNIT($,.RADIAN.)
) ;
#86334=(
NAMED_UNIT(*)
SI_UNIT($,.STERADIAN.)
SOLID_ANGLE_UNIT()
) ;
#86337=SHAPE_DEFINITION_REPRESENTATION(#86362,#86453) ;
#86362=PRODUCT_DEFINITION_SHAPE('',$,#86479) ;
#86453=SHAPE_REPRESENTATION('',(#32773),#86307) ;
#86476=PRODUCT_DEFINITION_CONTEXT('part definition',#86553,'design') ;
#86479=PRODUCT_DEFINITION('Lid','Lid',#86504,#86476) ;
#86504=PRODUCT_DEFINITION_FORMATION('',$,#86557) ;
#86553=APPLICATION_CONTEXT(
'Core Data for Automotive Mechanical Design Process') ;
#86554=PRODUCT_CONTEXT('part definition',#86553,'mechanical') ;
#86557=PRODUCT('Lid','Lid',$,(#86554)) ;
#86581=PRESENTATION_STYLE_ASSIGNMENT((#86586)) ;
#86586=SURFACE_STYLE_USAGE(.BOTH.,#86591) ;
#86591=SURFACE_SIDE_STYLE('',(#86596)) ;
#86596=SURFACE_STYLE_FILL_AREA(#86601) ;
#86601=FILL_AREA_STYLE('Opaque(228,229,230)',(#86606)) ;
#86606=FILL_AREA_STYLE_COLOUR('Opaque(228,229,230)',#86611) ;
#86611=COLOUR_RGB('Opaque(228,229,230)', 0.09019608, 0.27058824, 0.51372549) ;
ENDSEC;
END-ISO-10303-21;
